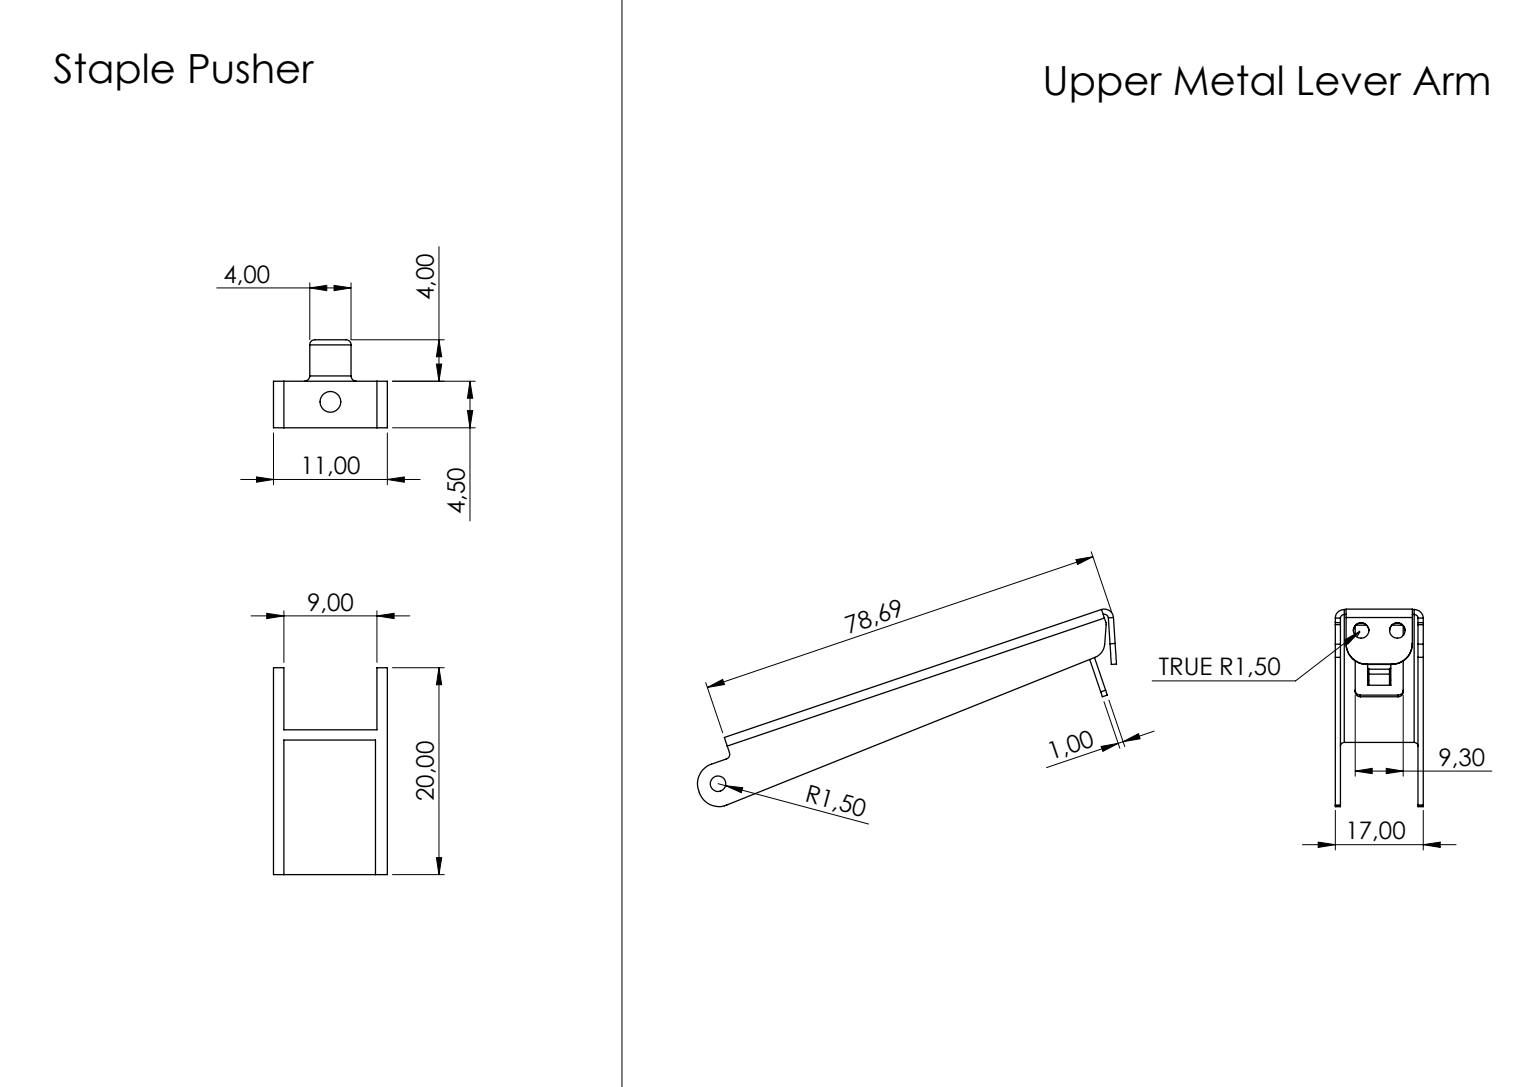
ISO-10303-21;
HEADER;
FILE_DESCRIPTION (('STEP AP214'),
    '1' );
FILE_NAME ('Staple Pusher.step',
    '2026-10-06T10:23:46',
    ( '' ),
    ( '' ),
    'SwSTEP 2.0',
    'SolidWorks 2020',
    '' );
FILE_SCHEMA (( 'AUTOMOTIVE_DESIGN' ));
ENDSEC;

DATA;
#63=ORIENTED_EDGE ( 'NONE', *, *, #7607, .F. ) ;
#105=( NAMED_UNIT ( * ) PLANE_ANGLE_UNIT ( ) SI_UNIT ( $, .RADIAN. ) );
#123=ADVANCED_FACE ( 'NONE', ( #785 ), #7110, .F. ) ;
#143=VECTOR ( 'NONE', #19074, 1000.000000000000000 ) ;
#190=ORIENTED_EDGE ( 'NONE', *, *, #18404, .F. ) ;
#193=DIRECTION ( 'NONE',  ( -1.927470528863119788E-16, -1.000000000000000000, 2.999999999999999839E-15 ) ) ;
#203=VERTEX_POINT ( 'NONE', #23192 ) ;
#209=LINE ( 'NONE', #23668, #17662 ) ;
#231=EDGE_CURVE ( 'NONE', #16465, #14577, #22942, .T. ) ;
#236=CARTESIAN_POINT ( 'NONE',  ( 40.81606138205700063, 9.191238522346999673, 69.30501292736997243 ) ) ;
#250=EDGE_CURVE ( 'NONE', #6034, #3058, #21270, .T. ) ;
#262=CARTESIAN_POINT ( 'NONE',  ( 32.81606138205700773, 2.191238522347013440, 73.80501292737000085 ) ) ;
#307=ORIENTED_EDGE ( 'NONE', *, *, #22779, .T. ) ;
#351=FACE_OUTER_BOUND ( 'NONE', #1891, .T. ) ;
#379=DIRECTION ( 'NONE',  ( 1.000000000000000000, 0.000000000000000000, 0.000000000000000000 ) ) ;
#383=AXIS2_PLACEMENT_3D ( 'NONE', #20572, #5122, #2903 ) ;
#385=CARTESIAN_POINT ( 'NONE',  ( 36.81606138205700063, 8.691238522346987239, 65.30501292736998664 ) ) ;
#404=EDGE_LOOP ( 'NONE', ( #18442, #12105, #307, #7710 ) ) ;
#415=ORIENTED_EDGE ( 'NONE', *, *, #6576, .T. ) ;
#419=CYLINDRICAL_SURFACE ( 'NONE', #8765, 0.5000000000000004441 ) ;
#442=ORIENTED_EDGE ( 'NONE', *, *, #7387, .T. ) ;
#462=DIRECTION ( 'NONE',  ( 1.000000000000000000, 3.614007241618344826E-17, -1.084202172485503317E-31 ) ) ;
#467=VERTEX_POINT ( 'NONE', #6689 ) ;
#486=PLANE ( 'NONE',  #5925 ) ;
#553=DIRECTION ( 'NONE',  ( 0.000000000000000000, 2.999999999999999839E-15, 1.000000000000000000 ) ) ;
#562=VERTEX_POINT ( 'NONE', #2686 ) ;
#577=ADVANCED_FACE ( 'NONE', ( #16345 ), #8767, .F. ) ;
#593=EDGE_CURVE ( 'NONE', #5442, #4334, #1137, .T. ) ;
#621=ORIENTED_EDGE ( 'NONE', *, *, #6367, .T. ) ;
#629=EDGE_LOOP ( 'NONE', ( #17511, #10756, #22625, #6939, #1629, #11779, #9994, #21905 ) ) ;
#650=EDGE_CURVE ( 'NONE', #5870, #848, #10535, .T. ) ;
#674=VECTOR ( 'NONE', #14592, 1000.000000000000000 ) ;
#690=CARTESIAN_POINT ( 'NONE',  ( 32.81606138205700773, 2.191238522347000117, 69.30501292737000085 ) ) ;
#728=DIRECTION ( 'NONE',  ( 0.000000000000000000, -1.000000000000000000, 2.999999999999999839E-15 ) ) ;
#732=( BOUNDED_CURVE ( )  B_SPLINE_CURVE ( 3, ( #2177, #11606, #21769, #236 ),
 .UNSPECIFIED., .F., .T. ) 
 B_SPLINE_CURVE_WITH_KNOTS ( ( 4, 4 ),
 ( 0.000000000000000000, 1.570796326794895004 ),
 .UNSPECIFIED. ) 
 CURVE ( )  GEOMETRIC_REPRESENTATION_ITEM ( )  RATIONAL_B_SPLINE_CURVE ( ( 1.000000000000000000, 0.8047378541243649375, 0.8047378541243649375, 1.000000000000000000 ) ) 
 REPRESENTATION_ITEM ( '' )  );
#761=CARTESIAN_POINT ( 'NONE',  ( 33.81606138205700063, 22.19123852234703520, 80.30501292736994401 ) ) ;
#785=FACE_OUTER_BOUND ( 'NONE', #18859, .T. ) ;
#797=VECTOR ( 'NONE', #6910, 1000.000000000000000 ) ;
#823=CARTESIAN_POINT ( 'NONE',  ( 36.31606138205700063, 8.691238522346989015, 65.80501292736998664 ) ) ;
#843=CARTESIAN_POINT ( 'NONE',  ( 40.31606138205700063, 8.691238522346987239, 65.30501292736998664 ) ) ;
#848=VERTEX_POINT ( 'NONE', #18891 ) ;
#858=DIRECTION ( 'NONE',  ( 0.000000000000000000, 2.999999999999999839E-15, 1.000000000000000000 ) ) ;
#900=EDGE_CURVE ( 'NONE', #13184, #17478, #14637, .T. ) ;
#904=VECTOR ( 'NONE', #2124, 1000.000000000000000 ) ;
#912=ADVANCED_FACE ( 'NONE', ( #16562 ), #11803, .T. ) ;
#927=LINE ( 'NONE', #12805, #16343 ) ;
#964=AXIS2_PLACEMENT_3D ( 'NONE', #21763, #4252, #7865 ) ;
#974=ORIENTED_EDGE ( 'NONE', *, *, #19644, .F. ) ;
#1000=VECTOR ( 'NONE', #20638, 1000.000000000000000 ) ;
#1001=CARTESIAN_POINT ( 'NONE',  ( 35.81606138205700063, 9.191238522346999673, 69.30501292736997243 ) ) ;
#1007=ORIENTED_EDGE ( 'NONE', *, *, #15153, .F. ) ;
#1092=EDGE_CURVE ( 'NONE', #467, #5442, #24144, .T. ) ;
#1096=DIRECTION ( 'NONE',  ( 0.000000000000000000, 1.000000000000000000, -2.999999999999999839E-15 ) ) ;
#1134=CARTESIAN_POINT ( 'NONE',  ( 33.81606138205700063, 15.19123852234700323, 70.30501292736995822 ) ) ;
#1137=LINE ( 'NONE', #2653, #13495 ) ;
#1179=DIRECTION ( 'NONE',  ( 0.000000000000000000, 1.000000000000000000, -2.999999999999999839E-15 ) ) ;
#1184=ADVANCED_FACE ( 'NONE', ( #6400 ), #19925, .T. ) ;
#1216=EDGE_LOOP ( 'NONE', ( #10411, #24861, #10562, #15495, #17319, #20995, #18206, #9644 ) ) ;
#1217=VECTOR ( 'NONE', #3864, 1000.000000000000000 ) ;
#1267=ORIENTED_EDGE ( 'NONE', *, *, #5167, .T. ) ;
#1275=ADVANCED_FACE ( 'NONE', ( #8845 ), #16686, .F. ) ;
#1303=ORIENTED_EDGE ( 'NONE', *, *, #4139, .F. ) ;
#1313=ORIENTED_EDGE ( 'NONE', *, *, #19104, .T. ) ;
#1337=CARTESIAN_POINT ( 'NONE',  ( 32.81606138205700773, 2.191238522347013440, 73.80501292737000085 ) ) ;
#1365=CARTESIAN_POINT ( 'NONE',  ( 32.81606138205700773, 2.191238522347013440, 73.80501292737000085 ) ) ;
#1435=LINE ( 'NONE', #16906, #1000 ) ;
#1489=EDGE_LOOP ( 'NONE', ( #16805, #24401, #621, #24675, #16930 ) ) ;
#1492=CARTESIAN_POINT ( 'NONE',  ( 42.81606138205700063, 16.19123852234703520, 80.30501292736995822 ) ) ;
#1496=PLANE ( 'NONE',  #16992 ) ;
#1569=ORIENTED_EDGE ( 'NONE', *, *, #14152, .T. ) ;
#1629=ORIENTED_EDGE ( 'NONE', *, *, #3717, .T. ) ;
#1678=SURFACE_STYLE_FILL_AREA ( #9947 ) ;
#1738=DIRECTION ( 'NONE',  ( 0.000000000000000000, -2.999999999999999839E-15, -1.000000000000000000 ) ) ;
#1805=ADVANCED_FACE ( 'NONE', ( #22575 ), #20906, .F. ) ;
#1829=ORIENTED_EDGE ( 'NONE', *, *, #2608, .T. ) ;
#1839=ORIENTED_EDGE ( 'NONE', *, *, #24052, .F. ) ;
#1853=ORIENTED_EDGE ( 'NONE', *, *, #1903, .F. ) ;
#1891=EDGE_LOOP ( 'NONE', ( #16584, #9694, #23122, #20814 ) ) ;
#1903=EDGE_CURVE ( 'NONE', #12694, #9681, #8685, .T. ) ;
#1906=EDGE_CURVE ( 'NONE', #10160, #8707, #24745, .T. ) ;
#1911=CARTESIAN_POINT ( 'NONE',  ( 36.31606138205700063, 5.691238522346989903, 65.80501292736998664 ) ) ;
#1930=CARTESIAN_POINT ( 'NONE',  ( 32.81606138205700773, 2.191238522347013440, 73.80501292737000085 ) ) ;
#1936=PRESENTATION_STYLE_ASSIGNMENT (( #13426 ) ) ;
#1981=DIRECTION ( 'NONE',  ( 1.000000000000000000, 0.000000000000000000, -0.000000000000000000 ) ) ;
#1983=EDGE_LOOP ( 'NONE', ( #14043, #19238, #19687, #25097 ) ) ;
#1986=VERTEX_POINT ( 'NONE', #25119 ) ;
#1996=CARTESIAN_POINT ( 'NONE',  ( 38.31606138205700063, 15.19123852234700323, 70.30501292736995822 ) ) ;
#1998=DIRECTION ( 'NONE',  ( 0.000000000000000000, -2.999999999999999839E-15, -1.000000000000000000 ) ) ;
#2000=AXIS2_PLACEMENT_3D ( 'NONE', #9286, #12766, #22537 ) ;
#2012=CARTESIAN_POINT ( 'NONE',  ( 32.81606138205700773, 22.19123852234701388, 73.80501292736992980 ) ) ;
#2015=DIRECTION ( 'NONE',  ( -1.000000000000000000, 0.000000000000000000, 0.000000000000000000 ) ) ;
#2044=PLANE ( 'NONE',  #16388 ) ;
#2052=ORIENTED_EDGE ( 'NONE', *, *, #22004, .F. ) ;
#2059=EDGE_LOOP ( 'NONE', ( #10504, #1303, #7748, #10759, #1267 ) ) ;
#2102=CARTESIAN_POINT ( 'NONE',  ( 36.10895460087045450, 5.484131741160450879, 69.30501292736998664 ) ) ;
#2109=MECHANICAL_DESIGN_GEOMETRIC_PRESENTATION_REPRESENTATION('',(#21879),#6646);
#2124=DIRECTION ( 'NONE',  ( 1.000000000000000000, 0.000000000000000000, -0.000000000000000000 ) ) ;
#2141=FACE_OUTER_BOUND ( 'NONE', #11810, .T. ) ;
#2173=CARTESIAN_POINT ( 'NONE',  ( 43.81606138205700063, 8.191238522346990791, 65.80501292736998664 ) ) ;
#2177=CARTESIAN_POINT ( 'NONE',  ( 40.31606138205700063, 8.691238522346997897, 68.80501292736998664 ) ) ;
#2184=EDGE_CURVE ( 'NONE', #4421, #25070, #3535, .T. ) ;
#2217=CARTESIAN_POINT ( 'NONE',  ( 40.52316816324353965, 5.484131741160450879, 69.30501292736998664 ) ) ;
#2224=LINE ( 'NONE', #4423, #8434 ) ;
#2261=DIRECTION ( 'NONE',  ( 1.000000000000000000, 0.000000000000000000, 0.000000000000000000 ) ) ;
#2293=SURFACE_STYLE_FILL_AREA ( #20953 ) ;
#2315=DIRECTION ( 'NONE',  ( 0.000000000000000000, 1.000000000000000000, -2.999999999999999839E-15 ) ) ;
#2317=CARTESIAN_POINT ( 'NONE',  ( 36.31606138205699352, 8.691238522346996120, 69.09790614618343341 ) ) ;
#2323=CARTESIAN_POINT ( 'NONE',  ( 36.81606138205700063, 6.191238522346988127, 65.30501292736998664 ) ) ;
#2333=DIRECTION ( 'NONE',  ( 0.000000000000000000, 1.000000000000000000, -2.999999999999999839E-15 ) ) ;
#2397=PLANE ( 'NONE',  #13514 ) ;
#2404=EDGE_CURVE ( 'NONE', #6235, #17478, #14094, .T. ) ;
#2443=AXIS2_PLACEMENT_3D ( 'NONE', #4060, #8182, #10241 ) ;
#2510=DIRECTION ( 'NONE',  ( 0.000000000000000000, -2.999999999999999839E-15, -1.000000000000000000 ) ) ;
#2577=DIRECTION ( 'NONE',  ( 1.000000000000000000, 0.000000000000000000, -0.000000000000000000 ) ) ;
#2608=EDGE_CURVE ( 'NONE', #9423, #562, #927, .T. ) ;
#2622=VECTOR ( 'NONE', #19427, 1000.000000000000000 ) ;
#2627=CARTESIAN_POINT ( 'NONE',  ( 36.31606138205699352, 8.691238522346985462, 65.51211970855652567 ) ) ;
#2652=CARTESIAN_POINT ( 'NONE',  ( 36.31606138205700063, 9.191238522346999673, 69.30501292736997243 ) ) ;
#2653=CARTESIAN_POINT ( 'NONE',  ( 32.81606138205700773, 22.19123852234699967, 69.30501292736994401 ) ) ;
#2686=CARTESIAN_POINT ( 'NONE',  ( 40.31606138205700063, 8.691238522346989015, 65.80501292736998664 ) ) ;
#2694=CARTESIAN_POINT ( 'NONE',  ( 42.68042513965293949, 15.19123852234701388, 73.80501292736995822 ) ) ;
#2711=ORIENTED_EDGE ( 'NONE', *, *, #14927, .F. ) ;
#2724=VERTEX_POINT ( 'NONE', #15354 ) ;
#2742=CARTESIAN_POINT ( 'NONE',  ( 36.31606138205700063, 8.691238522346989015, 65.80501292736998664 ) ) ;
#2771=VECTOR ( 'NONE', #18659, 1000.000000000000000 ) ;
#2782=CARTESIAN_POINT ( 'NONE',  ( 36.31606138205700063, 5.691238522346988127, 65.30501292736998664 ) ) ;
#2812=CARTESIAN_POINT ( 'NONE',  ( 32.81606138205700773, 22.19123852234699967, 69.30501292736994401 ) ) ;
#2866=CIRCLE ( 'NONE', #6186, 1.000000000000000888 ) ;
#2900=ORIENTED_EDGE ( 'NONE', *, *, #21220, .T. ) ;
#2903=DIRECTION ( 'NONE',  ( 1.000000000000000000, 0.000000000000000000, 0.000000000000000000 ) ) ;
#2928=VERTEX_POINT ( 'NONE', #2323 ) ;
#2967=ORIENTED_EDGE ( 'NONE', *, *, #1092, .T. ) ;
#3033=CARTESIAN_POINT ( 'NONE',  ( 33.81606138205700063, 22.19123852234699967, 69.30501292736994401 ) ) ;
#3035=FACE_OUTER_BOUND ( 'NONE', #20986, .T. ) ;
#3058=VERTEX_POINT ( 'NONE', #8642 ) ;
#3146=CARTESIAN_POINT ( 'NONE',  ( 40.31606138205700773, 8.691238522346985462, 65.51211970855652567 ) ) ;
#3205=EDGE_CURVE ( 'NONE', #848, #2928, #20946, .T. ) ;
#3237=VECTOR ( 'NONE', #3931, 1000.000000000000000 ) ;
#3248=DIRECTION ( 'NONE',  ( 0.000000000000000000, 1.000000000000000000, -2.999999999999999839E-15 ) ) ;
#3279=DIRECTION ( 'NONE',  ( -1.956963323498894821E-16, 1.000000000000000000, -2.999999999999999839E-15 ) ) ;
#3295=( NAMED_UNIT ( * ) PLANE_ANGLE_UNIT ( ) SI_UNIT ( $, .RADIAN. ) );
#3314=VERTEX_POINT ( 'NONE', #19072 ) ;
#3331=LINE ( 'NONE', #5532, #19828 ) ;
#3347=AXIS2_PLACEMENT_3D ( 'NONE', #20363, #2315, #379 ) ;
#3356=EDGE_LOOP ( 'NONE', ( #23510, #24602, #16175, #23690 ) ) ;
#3385=CARTESIAN_POINT ( 'NONE',  ( 33.81606138205700063, 2.191238522347003226, 70.30501292737000085 ) ) ;
#3409=ADVANCED_FACE ( 'NONE', ( #12370 ), #2044, .F. ) ;
#3425=DIRECTION ( 'NONE',  ( 0.000000000000000000, 2.999999999999999839E-15, 1.000000000000000000 ) ) ;
#3438=PLANE ( 'NONE',  #4644 ) ;
#3449=LINE ( 'NONE', #13494, #11858 ) ;
#3509=CARTESIAN_POINT ( 'NONE',  ( 42.81606138205700063, 22.19123852234699967, 69.30501292736994401 ) ) ;
#3535=LINE ( 'NONE', #5478, #22502 ) ;
#3540=CARTESIAN_POINT ( 'NONE',  ( 42.81606138205700063, 2.191238522347013884, 73.80501292737000085 ) ) ;
#3568=VECTOR ( 'NONE', #24239, 1000.000000000000000 ) ;
#3583=CARTESIAN_POINT ( 'NONE',  ( 43.81606138205700063, 2.191238522347000117, 69.30501292737000085 ) ) ;
#3680=ORIENTED_EDGE ( 'NONE', *, *, #9929, .F. ) ;
#3703=ORIENTED_EDGE ( 'NONE', *, *, #9232, .T. ) ;
#3717=EDGE_CURVE ( 'NONE', #5857, #7071, #209, .T. ) ;
#3739=CARTESIAN_POINT ( 'NONE',  ( 43.81606138205700063, 2.191238522346988127, 65.30501292737000085 ) ) ;
#3748=FILL_AREA_STYLE_COLOUR ( '', #14877 ) ;
#3829=DIRECTION ( 'NONE',  ( 0.000000000000000000, 2.999999999999999839E-15, 1.000000000000000000 ) ) ;
#3864=DIRECTION ( 'NONE',  ( 1.927470528863119788E-16, 1.000000000000000000, -2.999999999999999839E-15 ) ) ;
#3876=APPLICATION_CONTEXT ( 'automotive_design' ) ;
#3931=DIRECTION ( 'NONE',  ( 1.000000000000000000, 0.000000000000000000, -0.000000000000000000 ) ) ;
#3986=DIRECTION ( 'NONE',  ( 0.000000000000000000, 1.000000000000000000, -2.999999999999999839E-15 ) ) ;
#4021=VECTOR ( 'NONE', #6407, 1000.000000000000000 ) ;
#4039=VECTOR ( 'NONE', #8852, 1000.000000000000000 ) ;
#4060=CARTESIAN_POINT ( 'NONE',  ( 40.31606138205700063, 9.191238522346997897, 68.80501292736998664 ) ) ;
#4121=( NAMED_UNIT ( * ) SI_UNIT ( $, .STERADIAN. ) SOLID_ANGLE_UNIT ( ) );
#4131=ORIENTED_EDGE ( 'NONE', *, *, #2404, .F. ) ;
#4139=EDGE_CURVE ( 'NONE', #15007, #21826, #25055, .T. ) ;
#4153=EDGE_CURVE ( 'NONE', #8707, #4754, #8867, .T. ) ;
#4155=PLANE ( 'NONE',  #12494 ) ;
#4173=CARTESIAN_POINT ( 'NONE',  ( 42.68042513965293949, 2.191238522347003226, 70.30501292737000085 ) ) ;
#4180=CARTESIAN_POINT ( 'NONE',  ( 36.31606138205700063, 5.691238522346998785, 68.80501292736998664 ) ) ;
#4252=DIRECTION ( 'NONE',  ( 0.000000000000000000, 2.999999999999999839E-15, 1.000000000000000000 ) ) ;
#4282=EDGE_CURVE ( 'NONE', #19015, #5870, #21143, .T. ) ;
#4334=VERTEX_POINT ( 'NONE', #14111 ) ;
#4356=ORIENTED_EDGE ( 'NONE', *, *, #22779, .F. ) ;
#4373=CARTESIAN_POINT ( 'NONE',  ( 33.81606138205700063, 2.191238522347003226, 70.30501292737000085 ) ) ;
#4377=CARTESIAN_POINT ( 'NONE',  ( 42.68042513965293949, 2.191238522347003226, 70.30501292737000085 ) ) ;
#4411=DIRECTION ( 'NONE',  ( 1.000000000000000000, 0.000000000000000000, 0.000000000000000000 ) ) ;
#4421=VERTEX_POINT ( 'NONE', #18601 ) ;
#4423=CARTESIAN_POINT ( 'NONE',  ( 33.81606138205700063, 15.19123852234701388, 73.80501292736995822 ) ) ;
#4473=CARTESIAN_POINT ( 'NONE',  ( 40.31606138205700063, 8.691238522346987239, 65.30501292736998664 ) ) ;
#4478=CARTESIAN_POINT ( 'NONE',  ( 42.81606138205700063, 22.19123852234703520, 80.30501292736994401 ) ) ;
#4484=ORIENTED_EDGE ( 'NONE', *, *, #14301, .F. ) ;
#4491=VECTOR ( 'NONE', #11130, 1000.000000000000000 ) ;
#4500=LINE ( 'NONE', #4377, #9031 ) ;
#4524=VECTOR ( 'NONE', #9145, 1000.000000000000000 ) ;
#4553=DIRECTION ( 'NONE',  ( 1.000000000000000000, 0.000000000000000000, -0.000000000000000000 ) ) ;
#4556=AXIS2_PLACEMENT_3D ( 'NONE', #21742, #12479, #6415 ) ;
#4644=AXIS2_PLACEMENT_3D ( 'NONE', #1492, #193, #1738 ) ;
#4683=ORIENTED_EDGE ( 'NONE', *, *, #18404, .T. ) ;
#4733=ORIENTED_EDGE ( 'NONE', *, *, #2184, .F. ) ;
#4754=VERTEX_POINT ( 'NONE', #12164 ) ;
#4768=EDGE_CURVE ( 'NONE', #13664, #17658, #23623, .T. ) ;
#4773=LINE ( 'NONE', #10717, #17444 ) ;
#4798=DIRECTION ( 'NONE',  ( 0.000000000000000000, -2.999999999999999839E-15, -1.000000000000000000 ) ) ;
#4867=CARTESIAN_POINT ( 'NONE',  ( 32.81606138205700773, 22.19123852234699967, 69.30501292736994401 ) ) ;
#4892=VERTEX_POINT ( 'NONE', #22564 ) ;
#4902=DIRECTION ( 'NONE',  ( 0.000000000000000000, -2.999999999999999839E-15, -1.000000000000000000 ) ) ;
#4963=CARTESIAN_POINT ( 'NONE',  ( 40.31606138205700063, 8.691238522346989015, 65.80501292736998664 ) ) ;
#5122=DIRECTION ( 'NONE',  ( 0.000000000000000000, 1.000000000000000000, -2.999999999999999839E-15 ) ) ;
#5130=AXIS2_PLACEMENT_3D ( 'NONE', #11785, #4553, #8421 ) ;
#5139=LINE ( 'NONE', #12749, #22298 ) ;
#5144=CARTESIAN_POINT ( 'NONE',  ( 32.81606138205700773, 22.19123852234701388, 73.80501292736992980 ) ) ;
#5166=ADVANCED_FACE ( 'NONE', ( #25104 ), #13541, .T. ) ;
#5167=EDGE_CURVE ( 'NONE', #22981, #13614, #2866, .T. ) ;
#5180=ORIENTED_EDGE ( 'NONE', *, *, #250, .T. ) ;
#5193=FACE_OUTER_BOUND ( 'NONE', #629, .T. ) ;
#5270=CARTESIAN_POINT ( 'NONE',  ( 40.31606138205700063, 5.191238522346999673, 69.30501292736998664 ) ) ;
#5397=UNCERTAINTY_MEASURE_WITH_UNIT (LENGTH_MEASURE( 1.000000000000000082E-05 ), #23294, 'distance_accuracy_value', 'NONE');
#5398=VECTOR ( 'NONE', #19032, 1000.000000000000000 ) ;
#5442=VERTEX_POINT ( 'NONE', #20474 ) ;
#5478=CARTESIAN_POINT ( 'NONE',  ( 32.81606138205700773, 16.19123852234701388, 73.80501292736995822 ) ) ;
#5485=EDGE_CURVE ( 'NONE', #6235, #15007, #12886, .T. ) ;
#5532=CARTESIAN_POINT ( 'NONE',  ( 33.81606138205700063, 2.191238522347013440, 73.80501292737000085 ) ) ;
#5623=EDGE_LOOP ( 'NONE', ( #15814, #4131, #21557, #25354 ) ) ;
#5631=FACE_OUTER_BOUND ( 'NONE', #13241, .T. ) ;
#5660=SURFACE_STYLE_USAGE ( .BOTH. , #25348 ) ;
#5661=CARTESIAN_POINT ( 'NONE',  ( 36.81606138205700063, 6.191238522346988127, 65.30501292736998664 ) ) ;
#5687=( NAMED_UNIT ( * ) PLANE_ANGLE_UNIT ( ) SI_UNIT ( $, .RADIAN. ) );
#5797=CARTESIAN_POINT ( 'NONE',  ( 42.68042513965293949, 2.191238522347013440, 73.80501292737000085 ) ) ;
#5844=PLANE ( 'NONE',  #5130 ) ;
#5857=VERTEX_POINT ( 'NONE', #690 ) ;
#5870=VERTEX_POINT ( 'NONE', #823 ) ;
#5886=LINE ( 'NONE', #7693, #23529 ) ;
#5925=AXIS2_PLACEMENT_3D ( 'NONE', #7171, #13095, #20823 ) ;
#5970=ORIENTED_EDGE ( 'NONE', *, *, #6000, .T. ) ;
#6000=EDGE_CURVE ( 'NONE', #10377, #3314, #16803, .T. ) ;
#6029=APPLICATION_CONTEXT ( 'automotive_design' ) ;
#6034=VERTEX_POINT ( 'NONE', #1337 ) ;
#6115=EDGE_LOOP ( 'NONE', ( #3703, #4356, #24721, #1853 ) ) ;
#6118=CARTESIAN_POINT ( 'NONE',  ( 42.81606138205700063, 16.19123852234703520, 80.30501292736995822 ) ) ;
#6137=LINE ( 'NONE', #24019, #24716 ) ;
#6141=CARTESIAN_POINT ( 'NONE',  ( 33.81606138205700063, 15.19123852234700323, 70.30501292736995822 ) ) ;
#6142=DIRECTION ( 'NONE',  ( 0.000000000000000000, -1.000000000000000000, 0.000000000000000000 ) ) ;
#6150=LINE ( 'NONE', #4473, #4021 ) ;
#6186=AXIS2_PLACEMENT_3D ( 'NONE', #23576, #21649, #11878 ) ;
#6188=ADVANCED_FACE ( 'NONE', ( #23480 ), #5844, .F. ) ;
#6202=DIRECTION ( 'NONE',  ( 0.000000000000000000, -1.000000000000000000, 2.999999999999999839E-15 ) ) ;
#6235=VERTEX_POINT ( 'NONE', #20134 ) ;
#6319=EDGE_CURVE ( 'NONE', #17478, #203, #2224, .T. ) ;
#6331=DIRECTION ( 'NONE',  ( 0.000000000000000000, -1.000000000000000000, 2.999999999999999839E-15 ) ) ;
#6367=EDGE_CURVE ( 'NONE', #13507, #6369, #1435, .T. ) ;
#6369=VERTEX_POINT ( 'NONE', #22568 ) ;
#6389=ORIENTED_EDGE ( 'NONE', *, *, #3205, .T. ) ;
#6400=FACE_OUTER_BOUND ( 'NONE', #10407, .T. ) ;
#6407=DIRECTION ( 'NONE',  ( 0.000000000000000000, 2.999999999999999839E-15, 1.000000000000000000 ) ) ;
#6415=DIRECTION ( 'NONE',  ( -1.445602896647339903E-16, 1.000000000000000000, -2.999999999999999839E-15 ) ) ;
#6416=EDGE_LOOP ( 'NONE', ( #15821, #22360, #20683, #13474 ) ) ;
#6455=CARTESIAN_POINT ( 'NONE',  ( 35.81606138205700063, 9.191238522346999673, 69.30501292736997243 ) ) ;
#6465=VECTOR ( 'NONE', #2510, 1000.000000000000000 ) ;
#6493=FACE_OUTER_BOUND ( 'NONE', #11204, .T. ) ;
#6518=ORIENTED_EDGE ( 'NONE', *, *, #16824, .F. ) ;
#6576=EDGE_CURVE ( 'NONE', #6034, #10160, #13422, .T. ) ;
#6646=( GEOMETRIC_REPRESENTATION_CONTEXT ( 3 ) GLOBAL_UNCERTAINTY_ASSIGNED_CONTEXT ( ( #16158 ) ) GLOBAL_UNIT_ASSIGNED_CONTEXT ( ( #25249, #5687, #23585 ) ) REPRESENTATION_CONTEXT ( 'NONE', 'WORKASPACE' ) );
#6647=LINE ( 'NONE', #14382, #6913 ) ;
#6655=VECTOR ( 'NONE', #13137, 1000.000000000000000 ) ;
#6689=CARTESIAN_POINT ( 'NONE',  ( 42.81606138205700063, 22.19123852234701388, 73.80501292736992980 ) ) ;
#6697=CARTESIAN_POINT ( 'NONE',  ( 36.81606138205700063, 2.191238522346989903, 65.80501292737000085 ) ) ;
#6771=ADVANCED_BREP_SHAPE_REPRESENTATION ( '', ( #17330, #2000 ), #23998 ) ;
#6894=DIRECTION ( 'NONE',  ( -1.000000000000000000, -1.956963323498894821E-16, 5.870889970496684443E-31 ) ) ;
#6910=DIRECTION ( 'NONE',  ( 0.000000000000000000, 1.000000000000000000, -2.999999999999999839E-15 ) ) ;
#6913=VECTOR ( 'NONE', #14508, 1000.000000000000000 ) ;
#6917=ORIENTED_EDGE ( 'NONE', *, *, #7387, .F. ) ;
#6924=EDGE_LOOP ( 'NONE', ( #11359, #2052 ) ) ;
#6928=EDGE_CURVE ( 'NONE', #13507, #203, #13012, .T. ) ;
#6939=ORIENTED_EDGE ( 'NONE', *, *, #18851, .F. ) ;
#6941=CARTESIAN_POINT ( 'NONE',  ( 40.31606138205700773, 5.691238522346986350, 65.51211970855653988 ) ) ;
#7016=DIRECTION ( 'NONE',  ( 0.000000000000000000, 1.000000000000000000, -2.999999999999999839E-15 ) ) ;
#7071=VERTEX_POINT ( 'NONE', #15696 ) ;
#7110=CYLINDRICAL_SURFACE ( 'NONE', #16342, 0.4999999999999995559 ) ;
#7171=CARTESIAN_POINT ( 'NONE',  ( 32.81606138205700773, 22.19123852234699967, 69.30501292736994401 ) ) ;
#7233=DIRECTION ( 'NONE',  ( 0.000000000000000000, 1.000000000000000000, -2.999999999999999839E-15 ) ) ;
#7244=CARTESIAN_POINT ( 'NONE',  ( 40.81606138205700063, 8.691238522346999673, 69.30501292736998664 ) ) ;
#7252=VECTOR ( 'NONE', #24084, 1000.000000000000000 ) ;
#7264=ORIENTED_EDGE ( 'NONE', *, *, #4282, .T. ) ;
#7300=DIRECTION ( 'NONE',  ( 1.000000000000000000, 0.000000000000000000, -0.000000000000000000 ) ) ;
#7316=CLOSED_SHELL ( 'NONE', ( #21757, #912, #6188, #1275, #3409, #12132, #123, #21257, #11449, #9745, #1184, #13040, #8158, #5166, #24270, #17690, #19312, #24499, #19394, #14924, #1805, #12499, #9959, #577, #12730, #8926, #13194, #13060, #17434 ) ) ;
#7387=EDGE_CURVE ( 'NONE', #203, #3058, #16579, .T. ) ;
#7391=LINE ( 'NONE', #3385, #4491 ) ;
#7607=EDGE_CURVE ( 'NONE', #4892, #2928, #5886, .T. ) ;
#7693=CARTESIAN_POINT ( 'NONE',  ( 36.31606138205700063, 6.191238522346988127, 65.30501292736998664 ) ) ;
#7710=ORIENTED_EDGE ( 'NONE', *, *, #17518, .T. ) ;
#7748=ORIENTED_EDGE ( 'NONE', *, *, #7774, .F. ) ;
#7764=PRODUCT_CONTEXT ( 'NONE', #3876, 'mechanical' ) ;
#7774=EDGE_CURVE ( 'NONE', #17636, #15007, #10383, .T. ) ;
#7820=CARTESIAN_POINT ( 'NONE',  ( 37.31606138205700063, 12.69123852234700678, 71.30501292736997243 ) ) ;
#7864=CARTESIAN_POINT ( 'NONE',  ( 36.31606138205699352, 5.691238522346986350, 65.51211970855653988 ) ) ;
#7865=DIRECTION ( 'NONE',  ( 1.000000000000000000, 0.000000000000000000, -0.000000000000000000 ) ) ;
#8058=EDGE_LOOP ( 'NONE', ( #22523, #13290, #11880, #4484 ) ) ;
#8110=AXIS2_PLACEMENT_3D ( 'NONE', #19995, #2333, #4411 ) ;
#8158=ADVANCED_FACE ( 'NONE', ( #12524 ), #23829, .T. ) ;
#8182=DIRECTION ( 'NONE',  ( -1.000000000000000000, 0.000000000000000000, 0.000000000000000000 ) ) ;
#8202=DIRECTION ( 'NONE',  ( 1.000000000000000000, 0.000000000000000000, -0.000000000000000000 ) ) ;
#8305=DIRECTION ( 'NONE',  ( 1.000000000000000000, 0.000000000000000000, 0.000000000000000000 ) ) ;
#8336=ORIENTED_EDGE ( 'NONE', *, *, #6319, .F. ) ;
#8353=PLANE ( 'NONE',  #18198 ) ;
#8397=LINE ( 'NONE', #16239, #7252 ) ;
#8414=ORIENTED_EDGE ( 'NONE', *, *, #17520, .T. ) ;
#8421=DIRECTION ( 'NONE',  ( 0.000000000000000000, 2.999999999999999839E-15, 1.000000000000000000 ) ) ;
#8434=VECTOR ( 'NONE', #10102, 1000.000000000000000 ) ;
#8435=CARTESIAN_POINT ( 'NONE',  ( 40.81606138205700063, 5.691238522346998785, 68.80501292736998664 ) ) ;
#8533=CARTESIAN_POINT ( 'NONE',  ( 37.31606138205700063, 15.19123852234700500, 71.30501292736995822 ) ) ;
#8541=DIRECTION ( 'NONE',  ( 0.000000000000000000, 1.000000000000000000, -2.999999999999999839E-15 ) ) ;
#8642=CARTESIAN_POINT ( 'NONE',  ( 33.81606138205700063, 2.191238522347013440, 73.80501292737000085 ) ) ;
#8660=VECTOR ( 'NONE', #25232, 1000.000000000000000 ) ;
#8685=LINE ( 'NONE', #16915, #674 ) ;
#8707=VERTEX_POINT ( 'NONE', #4867 ) ;
#8750=CARTESIAN_POINT ( 'NONE',  ( 40.31606138205700063, 5.691238522346988127, 65.30501292736998664 ) ) ;
#8765=AXIS2_PLACEMENT_3D ( 'NONE', #8435, #20021, #8305 ) ;
#8767=PLANE ( 'NONE',  #11032 ) ;
#8808=AXIS2_PLACEMENT_3D ( 'NONE', #2173, #11739, #23809 ) ;
#8845=FACE_OUTER_BOUND ( 'NONE', #10900, .T. ) ;
#8852=DIRECTION ( 'NONE',  ( 0.000000000000000000, -2.999999999999999839E-15, -1.000000000000000000 ) ) ;
#8857=LINE ( 'NONE', #3033, #797 ) ;
#8867=LINE ( 'NONE', #20831, #17679 ) ;
#8913=ORIENTED_EDGE ( 'NONE', *, *, #1092, .F. ) ;
#8926=ADVANCED_FACE ( 'NONE', ( #5193 ), #13051, .F. ) ;
#8943=LINE ( 'NONE', #14353, #25032 ) ;
#8981=DIRECTION ( 'NONE',  ( -1.000000000000000000, 0.000000000000000000, 0.000000000000000000 ) ) ;
#8985=DIRECTION ( 'NONE',  ( 0.000000000000000000, -2.999999999999999839E-15, -1.000000000000000000 ) ) ;
#9031=VECTOR ( 'NONE', #20083, 1000.000000000000000 ) ;
#9099=CARTESIAN_POINT ( 'NONE',  ( 40.10895460087045450, 8.484131741160446438, 65.30501292736998664 ) ) ;
#9141=CARTESIAN_POINT ( 'NONE',  ( 36.81606138205700063, 8.191238522346989015, 65.30501292736998664 ) ) ;
#9145=DIRECTION ( 'NONE',  ( 1.000000000000000000, 0.000000000000000000, -0.000000000000000000 ) ) ;
#9232=EDGE_CURVE ( 'NONE', #12694, #22231, #24566, .T. ) ;
#9264=EDGE_CURVE ( 'NONE', #562, #5870, #8397, .T. ) ;
#9286=CARTESIAN_POINT ( 'NONE',  ( 0.000000000000000000, 0.000000000000000000, 0.000000000000000000 ) ) ;
#9423=VERTEX_POINT ( 'NONE', #16615 ) ;
#9567=VECTOR ( 'NONE', #23708, 1000.000000000000000 ) ;
#9636=CARTESIAN_POINT ( 'NONE',  ( 32.81606138205700773, 22.19123852234701388, 73.80501292736992980 ) ) ;
#9640=MECHANICAL_DESIGN_GEOMETRIC_PRESENTATION_REPRESENTATION('',(#17438),#12526);
#9644=ORIENTED_EDGE ( 'NONE', *, *, #15572, .F. ) ;
#9652=PLANE ( 'NONE',  #10635 ) ;
#9653=PRODUCT_DEFINITION ( 'UNKNOWN', '', #23210, #16222 ) ;
#9681=VERTEX_POINT ( 'NONE', #20078 ) ;
#9694=ORIENTED_EDGE ( 'NONE', *, *, #2608, .F. ) ;
#9705=PLANE ( 'NONE',  #18258 ) ;
#9745=ADVANCED_FACE ( 'NONE', ( #351 ), #10164, .T. ) ;
#9814=DIRECTION ( 'NONE',  ( 1.000000000000000000, 0.000000000000000000, -0.000000000000000000 ) ) ;
#9897=CYLINDRICAL_SURFACE ( 'NONE', #14910, 0.5000000000000004441 ) ;
#9929=EDGE_CURVE ( 'NONE', #848, #9423, #23141, .T. ) ;
#9947=FILL_AREA_STYLE ('',( #3748 ) ) ;
#9959=ADVANCED_FACE ( 'NONE', ( #5631 ), #1496, .T. ) ;
#9963=VECTOR ( 'NONE', #6331, 1000.000000000000000 ) ;
#9994=ORIENTED_EDGE ( 'NONE', *, *, #17987, .F. ) ;
#10024=DIRECTION ( 'NONE',  ( 0.000000000000000000, 2.999999999999999839E-15, 1.000000000000000000 ) ) ;
#10097=CARTESIAN_POINT ( 'NONE',  ( 40.31606138205700063, 5.691238522346998785, 68.80501292736998664 ) ) ;
#10102=DIRECTION ( 'NONE',  ( -1.000000000000000000, -1.956963323498894821E-16, 5.870889970496684443E-31 ) ) ;
#10131=DIRECTION ( 'NONE',  ( 0.000000000000000000, 1.000000000000000000, -2.999999999999999839E-15 ) ) ;
#10160=VERTEX_POINT ( 'NONE', #2012 ) ;
#10164=CYLINDRICAL_SURFACE ( 'NONE', #20689, 0.5000000000000004441 ) ;
#10208=VECTOR ( 'NONE', #11060, 1000.000000000000000 ) ;
#10239=LINE ( 'NONE', #6118, #16453 ) ;
#10241=DIRECTION ( 'NONE',  ( 0.000000000000000000, 1.000000000000000000, 0.000000000000000000 ) ) ;
#10368=ORIENTED_EDGE ( 'NONE', *, *, #9264, .T. ) ;
#10377=VERTEX_POINT ( 'NONE', #14875 ) ;
#10383=CIRCLE ( 'NONE', #19021, 1.000000000000000888 ) ;
#10391=ORIENTED_EDGE ( 'NONE', *, *, #1906, .T. ) ;
#10407=EDGE_LOOP ( 'NONE', ( #6389, #63, #1839, #3680 ) ) ;
#10411=ORIENTED_EDGE ( 'NONE', *, *, #4153, .T. ) ;
#10414=LINE ( 'NONE', #2782, #18194 ) ;
#10433=COLOUR_RGB ( '', 0.66274510, 0.83137255, 0.94901961) ;
#10489=ORIENTED_EDGE ( 'NONE', *, *, #18787, .F. ) ;
#10504=ORIENTED_EDGE ( 'NONE', *, *, #24901, .F. ) ;
#10519=CARTESIAN_POINT ( 'NONE',  ( 42.81606138205700063, 22.19123852234703520, 80.30501292736994401 ) ) ;
#10535=LINE ( 'NONE', #18012, #14714 ) ;
#10536=FACE_OUTER_BOUND ( 'NONE', #20667, .T. ) ;
#10562=ORIENTED_EDGE ( 'NONE', *, *, #231, .F. ) ;
#10573=AXIS2_PLACEMENT_3D ( 'NONE', #23899, #8202, #6142 ) ;
#10594=VECTOR ( 'NONE', #7300, 1000.000000000000000 ) ;
#10635=AXIS2_PLACEMENT_3D ( 'NONE', #25326, #21481, #3829 ) ;
#10716=EDGE_CURVE ( 'NONE', #20891, #19678, #13098, .T. ) ;
#10717=CARTESIAN_POINT ( 'NONE',  ( 33.81606138205700063, 2.191238522347003226, 70.30501292737000085 ) ) ;
#10730=DIRECTION ( 'NONE',  ( 1.000000000000000000, 0.000000000000000000, -0.000000000000000000 ) ) ;
#10756=ORIENTED_EDGE ( 'NONE', *, *, #20283, .T. ) ;
#10759=ORIENTED_EDGE ( 'NONE', *, *, #20936, .T. ) ;
#10804=LINE ( 'NONE', #8750, #2771 ) ;
#10824=VECTOR ( 'NONE', #12040, 1000.000000000000000 ) ;
#10900=EDGE_LOOP ( 'NONE', ( #21455, #23238, #1569, #20821, #12695, #19741, #21236, #24698 ) ) ;
#10912=PLANE ( 'NONE',  #11573 ) ;
#10951=ORIENTED_EDGE ( 'NONE', *, *, #25045, .T. ) ;
#10965=ORIENTED_EDGE ( 'NONE', *, *, #15849, .F. ) ;
#11032=AXIS2_PLACEMENT_3D ( 'NONE', #2812, #18673, #16604 ) ;
#11034=DIRECTION ( 'NONE',  ( 0.000000000000000000, 1.000000000000000000, -2.999999999999999839E-15 ) ) ;
#11060=DIRECTION ( 'NONE',  ( 0.000000000000000000, 1.000000000000000000, -2.999999999999999839E-15 ) ) ;
#11130=DIRECTION ( 'NONE',  ( 0.000000000000000000, 2.999999999999999839E-15, 1.000000000000000000 ) ) ;
#11204=EDGE_LOOP ( 'NONE', ( #19772, #10965, #13766, #190 ) ) ;
#11224=LINE ( 'NONE', #22806, #143 ) ;
#11310=EDGE_CURVE ( 'NONE', #5870, #12694, #5139, .T. ) ;
#11323=DIRECTION ( 'NONE',  ( 0.000000000000000000, 1.000000000000000000, -2.999999999999999839E-15 ) ) ;
#11351=FACE_OUTER_BOUND ( 'NONE', #11483, .T. ) ;
#11359=ORIENTED_EDGE ( 'NONE', *, *, #5167, .F. ) ;
#11382=DIRECTION ( 'NONE',  ( 3.614007241618344826E-17, -1.000000000000000000, 2.999999999999999839E-15 ) ) ;
#11449=ADVANCED_FACE ( 'NONE', ( #11708 ), #9897, .F. ) ;
#11483=EDGE_LOOP ( 'NONE', ( #7264, #24776, #6518, #11621 ) ) ;
#11485=LINE ( 'NONE', #13409, #23037 ) ;
#11573=AXIS2_PLACEMENT_3D ( 'NONE', #18764, #1096, #8985 ) ;
#11606=CARTESIAN_POINT ( 'NONE',  ( 40.31606138205700773, 8.691238522346996120, 69.09790614618343341 ) ) ;
#11619=DIRECTION ( 'NONE',  ( -1.000000000000000000, 1.927470528863119788E-16, -5.782411586589358909E-31 ) ) ;
#11621=ORIENTED_EDGE ( 'NONE', *, *, #19958, .F. ) ;
#11679=CARTESIAN_POINT ( 'NONE',  ( 39.31606138205700063, 16.19123852234700678, 71.30501292736995822 ) ) ;
#11705=DIRECTION ( 'NONE',  ( -1.000000000000000000, 0.000000000000000000, 0.000000000000000000 ) ) ;
#11708=FACE_OUTER_BOUND ( 'NONE', #22440, .T. ) ;
#11717=ORIENTED_EDGE ( 'NONE', *, *, #7607, .T. ) ;
#11739=DIRECTION ( 'NONE',  ( -1.000000000000000000, 0.000000000000000000, 0.000000000000000000 ) ) ;
#11755=ORIENTED_EDGE ( 'NONE', *, *, #14287, .F. ) ;
#11779=ORIENTED_EDGE ( 'NONE', *, *, #20081, .T. ) ;
#11785=CARTESIAN_POINT ( 'NONE',  ( 42.68042513965293949, 2.191238522347003226, 70.30501292737000085 ) ) ;
#11803=PLANE ( 'NONE',  #20865 ) ;
#11810=EDGE_LOOP ( 'NONE', ( #2967, #20673, #13703, #974 ) ) ;
#11836=VECTOR ( 'NONE', #11034, 1000.000000000000000 ) ;
#11840=EDGE_LOOP ( 'NONE', ( #16477, #24634, #10489, #4733 ) ) ;
#11858=VECTOR ( 'NONE', #16983, 1000.000000000000000 ) ;
#11878=DIRECTION ( 'NONE',  ( 1.000000000000000000, 0.000000000000000000, 0.000000000000000000 ) ) ;
#11880=ORIENTED_EDGE ( 'NONE', *, *, #17520, .F. ) ;
#11998=LINE ( 'NONE', #13661, #1217 ) ;
#12032=ORIENTED_EDGE ( 'NONE', *, *, #18714, .T. ) ;
#12040=DIRECTION ( 'NONE',  ( 0.000000000000000000, 2.999999999999999839E-15, 1.000000000000000000 ) ) ;
#12047=EDGE_LOOP ( 'NONE', ( #21140, #8913, #14740, #10951 ) ) ;
#12105=ORIENTED_EDGE ( 'NONE', *, *, #15849, .T. ) ;
#12120=VECTOR ( 'NONE', #7016, 1000.000000000000000 ) ;
#12132=ADVANCED_FACE ( 'NONE', ( #6493 ), #419, .F. ) ;
#12159=CYLINDRICAL_SURFACE ( 'NONE', #8110, 1.000000000000000888 ) ;
#12164=CARTESIAN_POINT ( 'NONE',  ( 33.81606138205700063, 22.19123852234699967, 69.30501292736994401 ) ) ;
#12218=PLANE ( 'NONE',  #4556 ) ;
#12219=ORIENTED_EDGE ( 'NONE', *, *, #18983, .T. ) ;
#12224=DIRECTION ( 'NONE',  ( 0.000000000000000000, 2.999999999999999839E-15, 1.000000000000000000 ) ) ;
#12308=DIRECTION ( 'NONE',  ( 0.000000000000000000, -2.999999999999999839E-15, -1.000000000000000000 ) ) ;
#12329=CARTESIAN_POINT ( 'NONE',  ( 33.81606138205700063, 16.19123852234701388, 73.80501292736995822 ) ) ;
#12370=FACE_OUTER_BOUND ( 'NONE', #15620, .T. ) ;
#12409=ORIENTED_EDGE ( 'NONE', *, *, #19958, .T. ) ;
#12439=EDGE_CURVE ( 'NONE', #5442, #16465, #17556, .T. ) ;
#12479=DIRECTION ( 'NONE',  ( -1.000000000000000000, -1.445602896647339903E-16, 4.336808689942019400E-31 ) ) ;
#12494=AXIS2_PLACEMENT_3D ( 'NONE', #262, #4902, #16360 ) ;
#12499=ADVANCED_FACE ( 'NONE', ( #21168 ), #9705, .F. ) ;
#12524=FACE_OUTER_BOUND ( 'NONE', #3356, .T. ) ;
#12526=( GEOMETRIC_REPRESENTATION_CONTEXT ( 3 ) GLOBAL_UNCERTAINTY_ASSIGNED_CONTEXT ( ( #5397 ) ) GLOBAL_UNIT_ASSIGNED_CONTEXT ( ( #23294, #105, #4121 ) ) REPRESENTATION_CONTEXT ( 'NONE', 'WORKASPACE' ) );
#12579=CARTESIAN_POINT ( 'NONE',  ( 37.31606138205700063, 16.19123852234700678, 71.30501292736995822 ) ) ;
#12673=CARTESIAN_POINT ( 'NONE',  ( 38.31606138205700063, 15.19123852234700500, 71.30501292736995822 ) ) ;
#12694=VERTEX_POINT ( 'NONE', #23966 ) ;
#12695=ORIENTED_EDGE ( 'NONE', *, *, #5485, .F. ) ;
#12730=ADVANCED_FACE ( 'NONE', ( #13940 ), #4155, .F. ) ;
#12749=CARTESIAN_POINT ( 'NONE',  ( 36.31606138205700063, 8.691238522346987239, 65.30501292736998664 ) ) ;
#12757=CARTESIAN_POINT ( 'NONE',  ( 40.31606138205700063, 5.691238522346989903, 65.80501292736998664 ) ) ;
#12766=DIRECTION ( 'NONE',  ( 0.000000000000000000, 0.000000000000000000, 1.000000000000000000 ) ) ;
#12805=CARTESIAN_POINT ( 'NONE',  ( 40.31606138205700063, 8.691238522346989015, 65.80501292736998664 ) ) ;
#12866=EDGE_CURVE ( 'NONE', #6369, #16802, #4773, .T. ) ;
#12886=LINE ( 'NONE', #1134, #24293 ) ;
#12977=CARTESIAN_POINT ( 'NONE',  ( 42.68042513965293949, 2.191238522347013440, 73.80501292737000085 ) ) ;
#13012=LINE ( 'NONE', #14553, #21207 ) ;
#13023=EDGE_CURVE ( 'NONE', #15007, #13507, #11224, .T. ) ;
#13040=ADVANCED_FACE ( 'NONE', ( #11351 ), #15954, .T. ) ;
#13051=PLANE ( 'NONE',  #18405 ) ;
#13060=ADVANCED_FACE ( 'NONE', ( #15575, #21892 ), #15833, .F. ) ;
#13095=DIRECTION ( 'NONE',  ( 0.000000000000000000, -1.000000000000000000, 2.999999999999999839E-15 ) ) ;
#13098=( BOUNDED_CURVE ( )  B_SPLINE_CURVE ( 3, ( #19761, #2102, #17844, #4180 ),
 .UNSPECIFIED., .F., .T. ) 
 B_SPLINE_CURVE_WITH_KNOTS ( ( 4, 4 ),
 ( 1.570796326794895004, 3.141592653589795336 ),
 .UNSPECIFIED. ) 
 CURVE ( )  GEOMETRIC_REPRESENTATION_ITEM ( )  RATIONAL_B_SPLINE_CURVE ( ( 1.000000000000000000, 0.8047378541243649375, 0.8047378541243649375, 1.000000000000000000 ) ) 
 REPRESENTATION_ITEM ( '' )  );
#13137=DIRECTION ( 'NONE',  ( 1.000000000000000000, 0.000000000000000000, -0.000000000000000000 ) ) ;
#13184=VERTEX_POINT ( 'NONE', #5797 ) ;
#13186=DIRECTION ( 'NONE',  ( -1.445602896647339903E-16, 1.000000000000000000, -2.999999999999999839E-15 ) ) ;
#13194=ADVANCED_FACE ( 'NONE', ( #17527 ), #486, .F. ) ;
#13206=ORIENTED_EDGE ( 'NONE', *, *, #23492, .T. ) ;
#13232=( LENGTH_UNIT ( ) NAMED_UNIT ( * ) SI_UNIT ( .MILLI., .METRE. ) );
#13241=EDGE_LOOP ( 'NONE', ( #25082, #415, #10391, #23792 ) ) ;
#13242=FACE_OUTER_BOUND ( 'NONE', #11840, .T. ) ;
#13278=VECTOR ( 'NONE', #10131, 1000.000000000000000 ) ;
#13290=ORIENTED_EDGE ( 'NONE', *, *, #22858, .T. ) ;
#13390=ORIENTED_EDGE ( 'NONE', *, *, #11310, .T. ) ;
#13409=CARTESIAN_POINT ( 'NONE',  ( 39.81606138205699352, 5.691238522346988127, 65.30501292736998664 ) ) ;
#13422=LINE ( 'NONE', #17671, #20772 ) ;
#13426=SURFACE_STYLE_USAGE ( .BOTH. , #15600 ) ;
#13444=ORIENTED_EDGE ( 'NONE', *, *, #6367, .F. ) ;
#13468=LINE ( 'NONE', #3540, #19686 ) ;
#13474=ORIENTED_EDGE ( 'NONE', *, *, #6000, .F. ) ;
#13494=CARTESIAN_POINT ( 'NONE',  ( 40.31606138205700063, 5.691238522346998785, 68.80501292736998664 ) ) ;
#13495=VECTOR ( 'NONE', #20189, 1000.000000000000000 ) ;
#13496=CARTESIAN_POINT ( 'NONE',  ( 35.81606138205700063, 5.691238522346998785, 68.80501292736998664 ) ) ;
#13507=VERTEX_POINT ( 'NONE', #6141 ) ;
#13514=AXIS2_PLACEMENT_3D ( 'NONE', #4478, #462, #10024 ) ;
#13541=PLANE ( 'NONE',  #14007 ) ;
#13562=VECTOR ( 'NONE', #8981, 1000.000000000000000 ) ;
#13614=VERTEX_POINT ( 'NONE', #12579 ) ;
#13624=DIRECTION ( 'NONE',  ( 1.000000000000000000, 0.000000000000000000, -0.000000000000000000 ) ) ;
#13661=CARTESIAN_POINT ( 'NONE',  ( 39.31606138205700063, 12.69123852234700678, 71.30501292736997243 ) ) ;
#13664=VERTEX_POINT ( 'NONE', #20294 ) ;
#13703=ORIENTED_EDGE ( 'NONE', *, *, #23212, .F. ) ;
#13766=ORIENTED_EDGE ( 'NONE', *, *, #4768, .T. ) ;
#13940=FACE_OUTER_BOUND ( 'NONE', #19367, .T. ) ;
#14007=AXIS2_PLACEMENT_3D ( 'NONE', #3739, #15724, #15211 ) ;
#14034=PRESENTATION_STYLE_ASSIGNMENT (( #5660 ) ) ;
#14043=ORIENTED_EDGE ( 'NONE', *, *, #14152, .F. ) ;
#14094=LINE ( 'NONE', #18219, #3568 ) ;
#14111=CARTESIAN_POINT ( 'NONE',  ( 43.81606138205700063, 22.19123852234699967, 69.30501292736994401 ) ) ;
#14152=EDGE_CURVE ( 'NONE', #21826, #17636, #17834, .T. ) ;
#14221=DIRECTION ( 'NONE',  ( 0.000000000000000000, -1.000000000000000000, 2.999999999999999839E-15 ) ) ;
#14287=EDGE_CURVE ( 'NONE', #20891, #13664, #19299, .T. ) ;
#14291=ORIENTED_EDGE ( 'NONE', *, *, #14301, .T. ) ;
#14301=EDGE_CURVE ( 'NONE', #25070, #2724, #3331, .T. ) ;
#14330=CARTESIAN_POINT ( 'NONE',  ( 40.31606138205700773, 5.691238522346996120, 69.09790614618344762 ) ) ;
#14353=CARTESIAN_POINT ( 'NONE',  ( 43.81606138205700063, 2.191238522347000117, 69.30501292737000085 ) ) ;
#14382=CARTESIAN_POINT ( 'NONE',  ( 32.81606138205700773, 2.191238522347000117, 69.30501292737000085 ) ) ;
#14460=ORIENTED_EDGE ( 'NONE', *, *, #14600, .T. ) ;
#14491=ORIENTED_EDGE ( 'NONE', *, *, #9232, .F. ) ;
#14508=DIRECTION ( 'NONE',  ( 0.000000000000000000, 2.999999999999999839E-15, 1.000000000000000000 ) ) ;
#14553=CARTESIAN_POINT ( 'NONE',  ( 33.81606138205700063, 15.19123852234700323, 70.30501292736995822 ) ) ;
#14577=VERTEX_POINT ( 'NONE', #20331 ) ;
#14592=DIRECTION ( 'NONE',  ( 1.000000000000000000, 0.000000000000000000, -0.000000000000000000 ) ) ;
#14600=EDGE_CURVE ( 'NONE', #848, #19678, #10414, .T. ) ;
#14620=ORIENTED_EDGE ( 'NONE', *, *, #11310, .F. ) ;
#14637=LINE ( 'NONE', #12977, #11836 ) ;
#14670=DIRECTION ( 'NONE',  ( 0.000000000000000000, 2.999999999999999839E-15, 1.000000000000000000 ) ) ;
#14714=VECTOR ( 'NONE', #22114, 1000.000000000000000 ) ;
#14740=ORIENTED_EDGE ( 'NONE', *, *, #14927, .T. ) ;
#14772=DIRECTION ( 'NONE',  ( 1.000000000000000000, 0.000000000000000000, -0.000000000000000000 ) ) ;
#14874=ORIENTED_EDGE ( 'NONE', *, *, #10716, .T. ) ;
#14875=CARTESIAN_POINT ( 'NONE',  ( 43.81606138205700063, 2.191238522347013440, 73.80501292737000085 ) ) ;
#14877=COLOUR_RGB ( '', 0.66274510, 0.83137255, 0.94901961) ;
#14910=AXIS2_PLACEMENT_3D ( 'NONE', #13496, #21228, #2015 ) ;
#14924=ADVANCED_FACE ( 'NONE', ( #21093, #13242 ), #3438, .F. ) ;
#14927=EDGE_CURVE ( 'NONE', #467, #3314, #23512, .T. ) ;
#14958=CARTESIAN_POINT ( 'NONE',  ( 38.31606138205700063, 16.19123852234700678, 71.30501292736995822 ) ) ;
#15007=VERTEX_POINT ( 'NONE', #1996 ) ;
#15139=ORIENTED_EDGE ( 'NONE', *, *, #18714, .F. ) ;
#15153=EDGE_CURVE ( 'NONE', #19678, #12694, #20038, .T. ) ;
#15174=CARTESIAN_POINT ( 'NONE',  ( 39.81606138205699352, 6.191238522346988127, 65.30501292736998664 ) ) ;
#15211=DIRECTION ( 'NONE',  ( 0.000000000000000000, 1.000000000000000000, -2.999999999999999839E-15 ) ) ;
#15228=AXIS2_PLACEMENT_3D ( 'NONE', #6697, #6202, #18430 ) ;
#15230=SHAPE_DEFINITION_REPRESENTATION ( #17966, #15514 ) ;
#15331=LINE ( 'NONE', #23567, #8660 ) ;
#15354=CARTESIAN_POINT ( 'NONE',  ( 33.81606138205700063, 22.19123852234701388, 73.80501292736992980 ) ) ;
#15417=DIRECTION ( 'NONE',  ( -1.000000000000000000, -1.956963323498894821E-16, 5.870889970496684443E-31 ) ) ;
#15495=ORIENTED_EDGE ( 'NONE', *, *, #12439, .F. ) ;
#15514=SHAPE_REPRESENTATION ( 'Staple Pusher', ( #2000 ), #23998 ) ;
#15523=ORIENTED_EDGE ( 'NONE', *, *, #4153, .F. ) ;
#15539=DIRECTION ( 'NONE',  ( -1.000000000000000000, 0.000000000000000000, 0.000000000000000000 ) ) ;
#15572=EDGE_CURVE ( 'NONE', #8707, #5857, #20260, .T. ) ;
#15575=FACE_BOUND ( 'NONE', #404, .T. ) ;
#15583=ORIENTED_EDGE ( 'NONE', *, *, #17987, .T. ) ;
#15600=SURFACE_SIDE_STYLE ('',( #1678 ) ) ;
#15620=EDGE_LOOP ( 'NONE', ( #442, #18018, #13444, #19517 ) ) ;
#15631=EDGE_CURVE ( 'NONE', #16802, #13184, #16261, .T. ) ;
#15694=FILL_AREA_STYLE_COLOUR ( '', #10433 ) ;
#15696=CARTESIAN_POINT ( 'NONE',  ( 43.81606138205700063, 2.191238522347000117, 69.30501292737000085 ) ) ;
#15724=DIRECTION ( 'NONE',  ( 0.000000000000000000, -2.999999999999999839E-15, -1.000000000000000000 ) ) ;
#15814=ORIENTED_EDGE ( 'NONE', *, *, #900, .T. ) ;
#15821=ORIENTED_EDGE ( 'NONE', *, *, #20081, .F. ) ;
#15833=PLANE ( 'NONE',  #964 ) ;
#15849=EDGE_CURVE ( 'NONE', #13664, #22879, #22694, .T. ) ;
#15954=CYLINDRICAL_SURFACE ( 'NONE', #8808, 0.5000000000000004441 ) ;
#16080=DIRECTION ( 'NONE',  ( -1.445602896647339903E-16, 1.000000000000000000, -2.999999999999999839E-15 ) ) ;
#16107=CARTESIAN_POINT ( 'NONE',  ( 36.31606138205700063, 8.691238522346997897, 68.80501292736998664 ) ) ;
#16127=DIRECTION ( 'NONE',  ( 1.000000000000000000, 0.000000000000000000, 0.000000000000000000 ) ) ;
#16158=UNCERTAINTY_MEASURE_WITH_UNIT (LENGTH_MEASURE( 1.000000000000000082E-05 ), #25249, 'distance_accuracy_value', 'NONE');
#16175=ORIENTED_EDGE ( 'NONE', *, *, #4282, .F. ) ;
#16222=PRODUCT_DEFINITION_CONTEXT ( 'detailed design', #6029, 'design' ) ;
#16239=CARTESIAN_POINT ( 'NONE',  ( 36.31606138205700063, 8.691238522346989015, 65.80501292736998664 ) ) ;
#16261=LINE ( 'NONE', #4173, #10824 ) ;
#16342=AXIS2_PLACEMENT_3D ( 'NONE', #20896, #10730, #20385 ) ;
#16343=VECTOR ( 'NONE', #13186, 1000.000000000000000 ) ;
#16345=FACE_OUTER_BOUND ( 'NONE', #12047, .T. ) ;
#16360=DIRECTION ( 'NONE',  ( 0.000000000000000000, 1.000000000000000000, -2.999999999999999839E-15 ) ) ;
#16388=AXIS2_PLACEMENT_3D ( 'NONE', #4373, #23933, #3986 ) ;
#16416=CARTESIAN_POINT ( 'NONE',  ( 36.31606138205700063, 8.691238522346997897, 68.80501292736998664 ) ) ;
#16434=CARTESIAN_POINT ( 'NONE',  ( 40.81606138205700063, 9.191238522346999673, 69.30501292736997243 ) ) ;
#16453=VECTOR ( 'NONE', #12308, 1000.000000000000000 ) ;
#16465=VERTEX_POINT ( 'NONE', #17643 ) ;
#16477=ORIENTED_EDGE ( 'NONE', *, *, #23212, .T. ) ;
#16489=( BOUNDED_CURVE ( )  B_SPLINE_CURVE ( 3, ( #12757, #6941, #19052, #15174 ),
 .UNSPECIFIED., .F., .T. ) 
 B_SPLINE_CURVE_WITH_KNOTS ( ( 4, 4 ),
 ( 0.000000000000000000, 1.570796326794895004 ),
 .UNSPECIFIED. ) 
 CURVE ( )  GEOMETRIC_REPRESENTATION_ITEM ( )  RATIONAL_B_SPLINE_CURVE ( ( 1.000000000000000000, 0.8047378541243649375, 0.8047378541243649375, 1.000000000000000000 ) ) 
 REPRESENTATION_ITEM ( '' )  );
#16508=EDGE_CURVE ( 'NONE', #4334, #7071, #23162, .T. ) ;
#16549=CARTESIAN_POINT ( 'NONE',  ( 33.81606138205700063, 15.19123852234700323, 70.30501292736995822 ) ) ;
#16562=FACE_OUTER_BOUND ( 'NONE', #1489, .T. ) ;
#16579=LINE ( 'NONE', #20454, #17810 ) ;
#16584=ORIENTED_EDGE ( 'NONE', *, *, #16824, .T. ) ;
#16604=DIRECTION ( 'NONE',  ( -1.000000000000000000, 0.000000000000000000, 0.000000000000000000 ) ) ;
#16615=CARTESIAN_POINT ( 'NONE',  ( 40.31606138205700063, 5.691238522346989903, 65.80501292736998664 ) ) ;
#16686=PLANE ( 'NONE',  #22098 ) ;
#16769=DIRECTION ( 'NONE',  ( -1.445602896647339903E-16, 1.000000000000000000, -2.999999999999999839E-15 ) ) ;
#16802=VERTEX_POINT ( 'NONE', #16809 ) ;
#16803=LINE ( 'NONE', #24636, #12120 ) ;
#16805=ORIENTED_EDGE ( 'NONE', *, *, #5485, .T. ) ;
#16809=CARTESIAN_POINT ( 'NONE',  ( 42.68042513965293949, 2.191238522347003226, 70.30501292737000085 ) ) ;
#16815=ORIENTED_EDGE ( 'NONE', *, *, #1903, .T. ) ;
#16824=EDGE_CURVE ( 'NONE', #1986, #562, #17334, .T. ) ;
#16906=CARTESIAN_POINT ( 'NONE',  ( 33.81606138205700063, 2.191238522347003226, 70.30501292737000085 ) ) ;
#16915=CARTESIAN_POINT ( 'NONE',  ( 40.31606138205700063, 8.691238522346997897, 68.80501292736998664 ) ) ;
#16930=ORIENTED_EDGE ( 'NONE', *, *, #22175, .T. ) ;
#16983=DIRECTION ( 'NONE',  ( 1.445602896647339903E-16, -1.000000000000000000, 2.999999999999999839E-15 ) ) ;
#16992=AXIS2_PLACEMENT_3D ( 'NONE', #21224, #11705, #11323 ) ;
#17005=VECTOR ( 'NONE', #14221, 1000.000000000000000 ) ;
#17009=CARTESIAN_POINT ( 'NONE',  ( 39.31606138205700063, 15.19123852234700500, 71.30501292736995822 ) ) ;
#17128=DIRECTION ( 'NONE',  ( 0.000000000000000000, 1.000000000000000000, -2.999999999999999839E-15 ) ) ;
#17210=DIRECTION ( 'NONE',  ( 3.614007241618344826E-17, -1.000000000000000000, 2.999999999999999839E-15 ) ) ;
#17319=ORIENTED_EDGE ( 'NONE', *, *, #593, .T. ) ;
#17330=MANIFOLD_SOLID_BREP ( 'NONE', #7316 ) ;
#17334=( BOUNDED_CURVE ( )  B_SPLINE_CURVE ( 3, ( #24518, #9099, #3146, #4963 ),
 .UNSPECIFIED., .F., .T. ) 
 B_SPLINE_CURVE_WITH_KNOTS ( ( 4, 4 ),
 ( 1.570796326794895004, 3.141592653589795336 ),
 .UNSPECIFIED. ) 
 CURVE ( )  GEOMETRIC_REPRESENTATION_ITEM ( )  RATIONAL_B_SPLINE_CURVE ( ( 1.000000000000000000, 0.8047378541243649375, 0.8047378541243649375, 1.000000000000000000 ) ) 
 REPRESENTATION_ITEM ( '' )  );
#17434=ADVANCED_FACE ( 'NONE', ( #24082 ), #23831, .F. ) ;
#17438=STYLED_ITEM ( 'NONE', ( #14034 ), #6771 ) ;
#17444=VECTOR ( 'NONE', #2577, 1000.000000000000000 ) ;
#17478=VERTEX_POINT ( 'NONE', #2694 ) ;
#17502=FACE_OUTER_BOUND ( 'NONE', #23990, .T. ) ;
#17511=ORIENTED_EDGE ( 'NONE', *, *, #12866, .F. ) ;
#17518=EDGE_CURVE ( 'NONE', #22231, #20891, #18431, .T. ) ;
#17520=EDGE_CURVE ( 'NONE', #2724, #4754, #18313, .T. ) ;
#17527=FACE_OUTER_BOUND ( 'NONE', #19189, .T. ) ;
#17556=LINE ( 'NONE', #3509, #24386 ) ;
#17624=AXIS2_PLACEMENT_3D ( 'NONE', #24364, #24484, #1179 ) ;
#17636=VERTEX_POINT ( 'NONE', #17009 ) ;
#17643=CARTESIAN_POINT ( 'NONE',  ( 42.81606138205700063, 16.19123852234699967, 69.30501292736995822 ) ) ;
#17658=VERTEX_POINT ( 'NONE', #22417 ) ;
#17662=VECTOR ( 'NONE', #23910, 1000.000000000000000 ) ;
#17671=CARTESIAN_POINT ( 'NONE',  ( 32.81606138205700773, 2.191238522347013440, 73.80501292737000085 ) ) ;
#17677=DIRECTION ( 'NONE',  ( 0.000000000000000000, -2.999999999999999839E-15, -1.000000000000000000 ) ) ;
#17679=VECTOR ( 'NONE', #14772, 1000.000000000000000 ) ;
#17688=FACE_OUTER_BOUND ( 'NONE', #2059, .T. ) ;
#17690=ADVANCED_FACE ( 'NONE', ( #22002 ), #8353, .F. ) ;
#17713=ORIENTED_EDGE ( 'NONE', *, *, #10716, .F. ) ;
#17715=DIRECTION ( 'NONE',  ( -1.000000000000000000, 1.927470528863119788E-16, -5.782411586589358909E-31 ) ) ;
#17810=VECTOR ( 'NONE', #728, 1000.000000000000000 ) ;
#17834=CIRCLE ( 'NONE', #21117, 1.000000000000000888 ) ;
#17844=CARTESIAN_POINT ( 'NONE',  ( 36.31606138205699352, 5.691238522346996120, 69.09790614618344762 ) ) ;
#17851=CARTESIAN_POINT ( 'NONE',  ( 40.31606138205700063, 8.191238522346989015, 65.30501292736998664 ) ) ;
#17966=PRODUCT_DEFINITION_SHAPE ( 'NONE', 'NONE',  #9653 ) ;
#17987=EDGE_CURVE ( 'NONE', #13184, #10377, #19026, .T. ) ;
#18010=VECTOR ( 'NONE', #11619, 1000.000000000000000 ) ;
#18012=CARTESIAN_POINT ( 'NONE',  ( 36.31606138205700063, 5.691238522346989903, 65.80501292736998664 ) ) ;
#18018=ORIENTED_EDGE ( 'NONE', *, *, #20283, .F. ) ;
#18032=CARTESIAN_POINT ( 'NONE',  ( 39.81606138205699352, 2.191238522346989015, 65.80501292737000085 ) ) ;
#18109=CYLINDRICAL_SURFACE ( 'NONE', #2443, 0.5000000000000004441 ) ;
#18194=VECTOR ( 'NONE', #12224, 1000.000000000000000 ) ;
#18198=AXIS2_PLACEMENT_3D ( 'NONE', #843, #20443, #24419 ) ;
#18204=CARTESIAN_POINT ( 'NONE',  ( 38.31606138205700063, 15.19123852234700500, 71.30501292736995822 ) ) ;
#18206=ORIENTED_EDGE ( 'NONE', *, *, #3717, .F. ) ;
#18219=CARTESIAN_POINT ( 'NONE',  ( 42.68042513965293949, 15.19123852234700323, 70.30501292736995822 ) ) ;
#18257=CARTESIAN_POINT ( 'NONE',  ( 33.81606138205700063, 16.19123852234703520, 80.30501292736995822 ) ) ;
#18258=AXIS2_PLACEMENT_3D ( 'NONE', #22964, #24877, #3248 ) ;
#18313=LINE ( 'NONE', #761, #9567 ) ;
#18376=LINE ( 'NONE', #18257, #4039 ) ;
#18404=EDGE_CURVE ( 'NONE', #9681, #17658, #3449, .T. ) ;
#18405=AXIS2_PLACEMENT_3D ( 'NONE', #20904, #21660, #17677 ) ;
#18430=DIRECTION ( 'NONE',  ( -1.000000000000000000, 0.000000000000000000, 0.000000000000000000 ) ) ;
#18431=LINE ( 'NONE', #20108, #9963 ) ;
#18442=ORIENTED_EDGE ( 'NONE', *, *, #14287, .T. ) ;
#18531=LINE ( 'NONE', #385, #10208 ) ;
#18601=CARTESIAN_POINT ( 'NONE',  ( 42.81606138205700063, 16.19123852234701388, 73.80501292736995822 ) ) ;
#18643=ORIENTED_EDGE ( 'NONE', *, *, #9929, .T. ) ;
#18659=DIRECTION ( 'NONE',  ( 0.000000000000000000, 2.999999999999999839E-15, 1.000000000000000000 ) ) ;
#18673=DIRECTION ( 'NONE',  ( 0.000000000000000000, -1.000000000000000000, 2.999999999999999839E-15 ) ) ;
#18714=EDGE_CURVE ( 'NONE', #562, #9681, #6150, .T. ) ;
#18764=CARTESIAN_POINT ( 'NONE',  ( 40.31606138205700063, 5.691238522346988127, 65.30501292736998664 ) ) ;
#18787=EDGE_CURVE ( 'NONE', #25070, #14577, #18376, .T. ) ;
#18851=EDGE_CURVE ( 'NONE', #5857, #6034, #6647, .T. ) ;
#18859=EDGE_LOOP ( 'NONE', ( #14874, #22019, #19012, #11755 ) ) ;
#18891=CARTESIAN_POINT ( 'NONE',  ( 36.31606138205700063, 5.691238522346989903, 65.80501292736998664 ) ) ;
#18983=EDGE_CURVE ( 'NONE', #2928, #19015, #18531, .T. ) ;
#19012=ORIENTED_EDGE ( 'NONE', *, *, #4768, .F. ) ;
#19015=VERTEX_POINT ( 'NONE', #9141 ) ;
#19021=AXIS2_PLACEMENT_3D ( 'NONE', #12673, #23775, #2261 ) ;
#19026=LINE ( 'NONE', #1365, #10594 ) ;
#19032=DIRECTION ( 'NONE',  ( 1.927470528863119788E-16, 1.000000000000000000, -2.999999999999999839E-15 ) ) ;
#19052=CARTESIAN_POINT ( 'NONE',  ( 40.10895460087045450, 5.898345303533535144, 65.30501292737000085 ) ) ;
#19055=UNCERTAINTY_MEASURE_WITH_UNIT (LENGTH_MEASURE( 1.000000000000000082E-05 ), #13232, 'distance_accuracy_value', 'NONE');
#19072=CARTESIAN_POINT ( 'NONE',  ( 43.81606138205700063, 22.19123852234701388, 73.80501292736992980 ) ) ;
#19074=DIRECTION ( 'NONE',  ( -1.000000000000000000, -1.956963323498894821E-16, 5.870889970496684443E-31 ) ) ;
#19085=DIRECTION ( 'NONE',  ( 1.000000000000000000, 0.000000000000000000, 0.000000000000000000 ) ) ;
#19104=EDGE_CURVE ( 'NONE', #9423, #17658, #10804, .T. ) ;
#19172=LINE ( 'NONE', #5144, #4524 ) ;
#19189=EDGE_LOOP ( 'NONE', ( #2900, #8414, #15523, #20554 ) ) ;
#19212=DIRECTION ( 'NONE',  ( 0.000000000000000000, 1.000000000000000000, -2.999999999999999839E-15 ) ) ;
#19238=ORIENTED_EDGE ( 'NONE', *, *, #24901, .T. ) ;
#19268=ORIENTED_EDGE ( 'NONE', *, *, #21220, .F. ) ;
#19299=LINE ( 'NONE', #5270, #6655 ) ;
#19312=ADVANCED_FACE ( 'NONE', ( #17502 ), #9652, .F. ) ;
#19367=EDGE_LOOP ( 'NONE', ( #5180, #6917, #8336, #22682, #15583, #5970, #2711, #22435, #22577, #14291, #19268, #20806 ) ) ;
#19375=PRODUCT ( 'Staple Pusher', 'Staple Pusher', '', ( #7764 ) ) ;
#19394=ADVANCED_FACE ( 'NONE', ( #2141 ), #2397, .F. ) ;
#19398=ORIENTED_EDGE ( 'NONE', *, *, #15153, .T. ) ;
#19427=DIRECTION ( 'NONE',  ( 0.000000000000000000, -1.000000000000000000, 2.999999999999999839E-15 ) ) ;
#19517=ORIENTED_EDGE ( 'NONE', *, *, #6928, .T. ) ;
#19589=CARTESIAN_POINT ( 'NONE',  ( 42.81606138205700063, 16.19123852234699967, 69.30501292736995822 ) ) ;
#19644=EDGE_CURVE ( 'NONE', #467, #4421, #13468, .T. ) ;
#19648=VECTOR ( 'NONE', #9814, 1000.000000000000000 ) ;
#19678=VERTEX_POINT ( 'NONE', #21079 ) ;
#19686=VECTOR ( 'NONE', #17210, 1000.000000000000000 ) ;
#19687=ORIENTED_EDGE ( 'NONE', *, *, #22004, .T. ) ;
#19741=ORIENTED_EDGE ( 'NONE', *, *, #2404, .T. ) ;
#19761=CARTESIAN_POINT ( 'NONE',  ( 35.81606138205700063, 5.191238522346999673, 69.30501292736998664 ) ) ;
#19767=ORIENTED_EDGE ( 'NONE', *, *, #19104, .F. ) ;
#19772=ORIENTED_EDGE ( 'NONE', *, *, #20895, .T. ) ;
#19828=VECTOR ( 'NONE', #17128, 1000.000000000000000 ) ;
#19870=VECTOR ( 'NONE', #16769, 1000.000000000000000 ) ;
#19878=CARTESIAN_POINT ( 'NONE',  ( 40.81606138205700063, 5.191238522346999673, 69.30501292736998664 ) ) ;
#19885=CARTESIAN_POINT ( 'NONE',  ( 32.81606138205700773, 2.191238522347000117, 69.30501292737000085 ) ) ;
#19906=FACE_OUTER_BOUND ( 'NONE', #6115, .T. ) ;
#19925=CYLINDRICAL_SURFACE ( 'NONE', #10573, 0.5000000000000004441 ) ;
#19958=EDGE_CURVE ( 'NONE', #19015, #1986, #22076, .T. ) ;
#19995=CARTESIAN_POINT ( 'NONE',  ( 38.31606138205700063, 12.69123852234700678, 71.30501292736997243 ) ) ;
#20021=DIRECTION ( 'NONE',  ( 0.000000000000000000, 1.000000000000000000, -2.999999999999999839E-15 ) ) ;
#20038=LINE ( 'NONE', #16416, #13278 ) ;
#20078=CARTESIAN_POINT ( 'NONE',  ( 40.31606138205700063, 8.691238522346997897, 68.80501292736998664 ) ) ;
#20081=EDGE_CURVE ( 'NONE', #7071, #10377, #8943, .T. ) ;
#20083=DIRECTION ( 'NONE',  ( 0.000000000000000000, 1.000000000000000000, -2.999999999999999839E-15 ) ) ;
#20108=CARTESIAN_POINT ( 'NONE',  ( 35.81606138205700063, 5.691238522347000561, 69.30501292736998664 ) ) ;
#20134=CARTESIAN_POINT ( 'NONE',  ( 42.68042513965293949, 15.19123852234700323, 70.30501292736995822 ) ) ;
#20189=DIRECTION ( 'NONE',  ( 1.000000000000000000, 0.000000000000000000, -0.000000000000000000 ) ) ;
#20244=ORIENTED_EDGE ( 'NONE', *, *, #17518, .F. ) ;
#20260=LINE ( 'NONE', #19885, #17005 ) ;
#20283=EDGE_CURVE ( 'NONE', #6369, #3058, #7391, .T. ) ;
#20292=CARTESIAN_POINT ( 'NONE',  ( 36.52316816324354676, 8.484131741160446438, 65.30501292736998664 ) ) ;
#20294=CARTESIAN_POINT ( 'NONE',  ( 40.81606138205700063, 5.191238522346999673, 69.30501292736998664 ) ) ;
#20331=CARTESIAN_POINT ( 'NONE',  ( 33.81606138205700063, 16.19123852234699967, 69.30501292736995822 ) ) ;
#20363=CARTESIAN_POINT ( 'NONE',  ( 38.31606138205700063, 12.69123852234700678, 71.30501292736997243 ) ) ;
#20385=DIRECTION ( 'NONE',  ( 0.000000000000000000, -1.000000000000000000, 0.000000000000000000 ) ) ;
#20443=DIRECTION ( 'NONE',  ( 0.000000000000000000, -1.000000000000000000, 2.999999999999999839E-15 ) ) ;
#20454=CARTESIAN_POINT ( 'NONE',  ( 33.81606138205700063, 2.191238522347013440, 73.80501292737000085 ) ) ;
#20474=CARTESIAN_POINT ( 'NONE',  ( 42.81606138205700063, 22.19123852234699967, 69.30501292736994401 ) ) ;
#20554=ORIENTED_EDGE ( 'NONE', *, *, #1906, .F. ) ;
#20572=CARTESIAN_POINT ( 'NONE',  ( 38.31606138205700063, 15.19123852234700500, 71.30501292736995822 ) ) ;
#20638=DIRECTION ( 'NONE',  ( 0.000000000000000000, -1.000000000000000000, 2.999999999999999839E-15 ) ) ;
#20667=EDGE_LOOP ( 'NONE', ( #19767, #1829, #12032, #4683 ) ) ;
#20673=ORIENTED_EDGE ( 'NONE', *, *, #12439, .T. ) ;
#20683=ORIENTED_EDGE ( 'NONE', *, *, #25045, .F. ) ;
#20689=AXIS2_PLACEMENT_3D ( 'NONE', #18032, #16080, #23929 ) ;
#20772=VECTOR ( 'NONE', #19212, 1000.000000000000000 ) ;
#20806=ORIENTED_EDGE ( 'NONE', *, *, #6576, .F. ) ;
#20814=ORIENTED_EDGE ( 'NONE', *, *, #23554, .F. ) ;
#20821=ORIENTED_EDGE ( 'NONE', *, *, #7774, .T. ) ;
#20823=DIRECTION ( 'NONE',  ( -1.000000000000000000, 0.000000000000000000, 0.000000000000000000 ) ) ;
#20831=CARTESIAN_POINT ( 'NONE',  ( 32.81606138205700773, 22.19123852234699967, 69.30501292736994401 ) ) ;
#20865=AXIS2_PLACEMENT_3D ( 'NONE', #23119, #3425, #1981 ) ;
#20879=ORIENTED_EDGE ( 'NONE', *, *, #650, .T. ) ;
#20891=VERTEX_POINT ( 'NONE', #22928 ) ;
#20895=EDGE_CURVE ( 'NONE', #9681, #22879, #732, .T. ) ;
#20896=CARTESIAN_POINT ( 'NONE',  ( 40.31606138205700063, 5.191238522346998785, 68.80501292736998664 ) ) ;
#20904=CARTESIAN_POINT ( 'NONE',  ( 32.81606138205700773, 2.191238522347000117, 69.30501292737000085 ) ) ;
#20906=PLANE ( 'NONE',  #17624 ) ;
#20936=EDGE_CURVE ( 'NONE', #17636, #22981, #11998, .T. ) ;
#20946=( BOUNDED_CURVE ( )  B_SPLINE_CURVE ( 3, ( #1911, #7864, #25349, #5661 ),
 .UNSPECIFIED., .F., .T. ) 
 B_SPLINE_CURVE_WITH_KNOTS ( ( 4, 4 ),
 ( 3.141592653589795336, 4.712388980384689674 ),
 .UNSPECIFIED. ) 
 CURVE ( )  GEOMETRIC_REPRESENTATION_ITEM ( )  RATIONAL_B_SPLINE_CURVE ( ( 1.000000000000000000, 0.8047378541243649375, 0.8047378541243649375, 1.000000000000000000 ) ) 
 REPRESENTATION_ITEM ( '' )  );
#20953=FILL_AREA_STYLE ('',( #15694 ) ) ;
#20960=CIRCLE ( 'NONE', #25026, 1.000000000000000888 ) ;
#20964=ORIENTED_EDGE ( 'NONE', *, *, #23554, .T. ) ;
#20986=EDGE_LOOP ( 'NONE', ( #21855, #18643, #1313, #13206 ) ) ;
#20995=ORIENTED_EDGE ( 'NONE', *, *, #16508, .T. ) ;
#21079=CARTESIAN_POINT ( 'NONE',  ( 36.31606138205700063, 5.691238522346998785, 68.80501292736998664 ) ) ;
#21093=FACE_BOUND ( 'NONE', #6924, .T. ) ;
#21101=CARTESIAN_POINT ( 'NONE',  ( 40.31606138205700063, 5.691238522346989903, 65.80501292736998664 ) ) ;
#21117=AXIS2_PLACEMENT_3D ( 'NONE', #18204, #8541, #16127 ) ;
#21140=ORIENTED_EDGE ( 'NONE', *, *, #593, .F. ) ;
#21143=( BOUNDED_CURVE ( )  B_SPLINE_CURVE ( 3, ( #22214, #20292, #2627, #2742 ),
 .UNSPECIFIED., .F., .T. ) 
 B_SPLINE_CURVE_WITH_KNOTS ( ( 4, 4 ),
 ( 1.570796326794895004, 3.141592653589795336 ),
 .UNSPECIFIED. ) 
 CURVE ( )  GEOMETRIC_REPRESENTATION_ITEM ( )  RATIONAL_B_SPLINE_CURVE ( ( 1.000000000000000000, 0.8047378541243649375, 0.8047378541243649375, 1.000000000000000000 ) ) 
 REPRESENTATION_ITEM ( '' )  );
#21168=FACE_OUTER_BOUND ( 'NONE', #6416, .T. ) ;
#21207=VECTOR ( 'NONE', #14670, 1000.000000000000000 ) ;
#21220=EDGE_CURVE ( 'NONE', #10160, #2724, #19172, .T. ) ;
#21224=CARTESIAN_POINT ( 'NONE',  ( 32.81606138205700773, 2.191238522347000117, 69.30501292737000085 ) ) ;
#21228=DIRECTION ( 'NONE',  ( 0.000000000000000000, -1.000000000000000000, 2.999999999999999839E-15 ) ) ;
#21236=ORIENTED_EDGE ( 'NONE', *, *, #6319, .T. ) ;
#21257=ADVANCED_FACE ( 'NONE', ( #19906 ), #18109, .F. ) ;
#21270=LINE ( 'NONE', #1930, #19648 ) ;
#21375=SHAPE_REPRESENTATION_RELATIONSHIP ( 'NONE' , 'NONE' ,  #15514, #6771 ) ;
#21455=ORIENTED_EDGE ( 'NONE', *, *, #13023, .F. ) ;
#21481=DIRECTION ( 'NONE',  ( 1.000000000000000000, 0.000000000000000000, -0.000000000000000000 ) ) ;
#21557=ORIENTED_EDGE ( 'NONE', *, *, #22175, .F. ) ;
#21649=DIRECTION ( 'NONE',  ( 0.000000000000000000, 1.000000000000000000, -2.999999999999999839E-15 ) ) ;
#21660=DIRECTION ( 'NONE',  ( 0.000000000000000000, 1.000000000000000000, -2.999999999999999839E-15 ) ) ;
#21742=CARTESIAN_POINT ( 'NONE',  ( 40.31606138205700063, 5.691238522346988127, 65.30501292736998664 ) ) ;
#21757=ADVANCED_FACE ( 'NONE', ( #17688 ), #12159, .F. ) ;
#21763=CARTESIAN_POINT ( 'NONE',  ( 32.81606138205700773, 2.191238522347000117, 69.30501292737000085 ) ) ;
#21769=CARTESIAN_POINT ( 'NONE',  ( 40.52316816324353965, 8.898345303533549355, 69.30501292736998664 ) ) ;
#21826=VERTEX_POINT ( 'NONE', #8533 ) ;
#21855=ORIENTED_EDGE ( 'NONE', *, *, #14600, .F. ) ;
#21879=STYLED_ITEM ( 'NONE', ( #1936 ), #17330 ) ;
#21892=FACE_OUTER_BOUND ( 'NONE', #1216, .T. ) ;
#21905=ORIENTED_EDGE ( 'NONE', *, *, #15631, .F. ) ;
#22002=FACE_OUTER_BOUND ( 'NONE', #23628, .T. ) ;
#22004=EDGE_CURVE ( 'NONE', #13614, #22981, #20960, .T. ) ;
#22019=ORIENTED_EDGE ( 'NONE', *, *, #23492, .F. ) ;
#22076=LINE ( 'NONE', #17851, #3237 ) ;
#22098=AXIS2_PLACEMENT_3D ( 'NONE', #16549, #3279, #6894 ) ;
#22114=DIRECTION ( 'NONE',  ( 0.000000000000000000, -1.000000000000000000, 2.999999999999999839E-15 ) ) ;
#22175=EDGE_CURVE ( 'NONE', #16802, #6235, #4500, .T. ) ;
#22214=CARTESIAN_POINT ( 'NONE',  ( 36.81606138205700063, 8.191238522346989015, 65.30501292736998664 ) ) ;
#22231=VERTEX_POINT ( 'NONE', #1001 ) ;
#22298=VECTOR ( 'NONE', #858, 1000.000000000000000 ) ;
#22360=ORIENTED_EDGE ( 'NONE', *, *, #16508, .F. ) ;
#22417=CARTESIAN_POINT ( 'NONE',  ( 40.31606138205700063, 5.691238522346998785, 68.80501292736998664 ) ) ;
#22435=ORIENTED_EDGE ( 'NONE', *, *, #19644, .T. ) ;
#22440=EDGE_LOOP ( 'NONE', ( #17713, #20244, #14491, #1007 ) ) ;
#22448=CARTESIAN_POINT ( 'NONE',  ( 32.81606138205700773, 22.19123852234699967, 69.30501292736994401 ) ) ;
#22502=VECTOR ( 'NONE', #17715, 1000.000000000000000 ) ;
#22523=ORIENTED_EDGE ( 'NONE', *, *, #18787, .T. ) ;
#22537=DIRECTION ( 'NONE',  ( 1.000000000000000000, 0.000000000000000000, 0.000000000000000000 ) ) ;
#22538=EDGE_LOOP ( 'NONE', ( #12409, #20964, #11717, #12219 ) ) ;
#22564=CARTESIAN_POINT ( 'NONE',  ( 39.81606138205699352, 6.191238522346988127, 65.30501292736998664 ) ) ;
#22568=CARTESIAN_POINT ( 'NONE',  ( 33.81606138205700063, 2.191238522347003226, 70.30501292737000085 ) ) ;
#22575=FACE_OUTER_BOUND ( 'NONE', #8058, .T. ) ;
#22577=ORIENTED_EDGE ( 'NONE', *, *, #2184, .T. ) ;
#22625=ORIENTED_EDGE ( 'NONE', *, *, #250, .F. ) ;
#22682=ORIENTED_EDGE ( 'NONE', *, *, #900, .F. ) ;
#22694=LINE ( 'NONE', #7244, #19870 ) ;
#22757=VECTOR ( 'NONE', #13624, 1000.000000000000000 ) ;
#22779=EDGE_CURVE ( 'NONE', #22879, #22231, #24039, .T. ) ;
#22806=CARTESIAN_POINT ( 'NONE',  ( 33.81606138205700063, 15.19123852234700323, 70.30501292736995822 ) ) ;
#22858=EDGE_CURVE ( 'NONE', #14577, #4754, #8857, .T. ) ;
#22879=VERTEX_POINT ( 'NONE', #16434 ) ;
#22928=CARTESIAN_POINT ( 'NONE',  ( 35.81606138205700063, 5.191238522346999673, 69.30501292736998664 ) ) ;
#22942=LINE ( 'NONE', #19589, #18010 ) ;
#22964=CARTESIAN_POINT ( 'NONE',  ( 43.81606138205700063, 2.191238522347000117, 69.30501292737000085 ) ) ;
#22981=VERTEX_POINT ( 'NONE', #11679 ) ;
#23037=VECTOR ( 'NONE', #23183, 1000.000000000000000 ) ;
#23119=CARTESIAN_POINT ( 'NONE',  ( 43.81606138205700063, 2.191238522347003226, 70.30501292737000085 ) ) ;
#23121=( NAMED_UNIT ( * ) SI_UNIT ( $, .STERADIAN. ) SOLID_ANGLE_UNIT ( ) );
#23122=ORIENTED_EDGE ( 'NONE', *, *, #24052, .T. ) ;
#23141=LINE ( 'NONE', #21101, #22757 ) ;
#23162=LINE ( 'NONE', #3583, #2622 ) ;
#23183=DIRECTION ( 'NONE',  ( 1.445602896647339903E-16, -1.000000000000000000, 2.999999999999999839E-15 ) ) ;
#23192=CARTESIAN_POINT ( 'NONE',  ( 33.81606138205700063, 15.19123852234701388, 73.80501292736995822 ) ) ;
#23210=PRODUCT_DEFINITION_FORMATION_WITH_SPECIFIED_SOURCE ( 'ANY', '', #19375, .NOT_KNOWN. ) ;
#23212=EDGE_CURVE ( 'NONE', #4421, #16465, #10239, .T. ) ;
#23238=ORIENTED_EDGE ( 'NONE', *, *, #4139, .T. ) ;
#23294=( LENGTH_UNIT ( ) NAMED_UNIT ( * ) SI_UNIT ( .MILLI., .METRE. ) );
#23480=FACE_OUTER_BOUND ( 'NONE', #5623, .T. ) ;
#23492=EDGE_CURVE ( 'NONE', #17658, #19678, #15331, .T. ) ;
#23510=ORIENTED_EDGE ( 'NONE', *, *, #3205, .F. ) ;
#23512=LINE ( 'NONE', #9636, #904 ) ;
#23529=VECTOR ( 'NONE', #15539, 1000.000000000000000 ) ;
#23554=EDGE_CURVE ( 'NONE', #1986, #4892, #11485, .T. ) ;
#23567=CARTESIAN_POINT ( 'NONE',  ( 36.31606138205700063, 5.691238522346998785, 68.80501292736998664 ) ) ;
#23576=CARTESIAN_POINT ( 'NONE',  ( 38.31606138205700063, 16.19123852234700678, 71.30501292736995822 ) ) ;
#23585=( NAMED_UNIT ( * ) SI_UNIT ( $, .STERADIAN. ) SOLID_ANGLE_UNIT ( ) );
#23623=( BOUNDED_CURVE ( )  B_SPLINE_CURVE ( 3, ( #19878, #2217, #14330, #10097 ),
 .UNSPECIFIED., .F., .T. ) 
 B_SPLINE_CURVE_WITH_KNOTS ( ( 4, 4 ),
 ( 1.570796326794895004, 3.141592653589795336 ),
 .UNSPECIFIED. ) 
 CURVE ( )  GEOMETRIC_REPRESENTATION_ITEM ( )  RATIONAL_B_SPLINE_CURVE ( ( 1.000000000000000000, 0.8047378541243649375, 0.8047378541243649375, 1.000000000000000000 ) ) 
 REPRESENTATION_ITEM ( '' )  );
#23628=EDGE_LOOP ( 'NONE', ( #15139, #10368, #13390, #16815 ) ) ;
#23668=CARTESIAN_POINT ( 'NONE',  ( 32.81606138205700773, 2.191238522347000117, 69.30501292737000085 ) ) ;
#23690=ORIENTED_EDGE ( 'NONE', *, *, #18983, .F. ) ;
#23708=DIRECTION ( 'NONE',  ( 0.000000000000000000, -2.999999999999999839E-15, -1.000000000000000000 ) ) ;
#23775=DIRECTION ( 'NONE',  ( 0.000000000000000000, 1.000000000000000000, -2.999999999999999839E-15 ) ) ;
#23792=ORIENTED_EDGE ( 'NONE', *, *, #15572, .T. ) ;
#23809=DIRECTION ( 'NONE',  ( 0.000000000000000000, 1.000000000000000000, 0.000000000000000000 ) ) ;
#23829=CYLINDRICAL_SURFACE ( 'NONE', #15228, 0.5000000000000004441 ) ;
#23831=CYLINDRICAL_SURFACE ( 'NONE', #3347, 1.000000000000000888 ) ;
#23899=CARTESIAN_POINT ( 'NONE',  ( 43.81606138205700063, 6.191238522346989903, 65.80501292736998664 ) ) ;
#23910=DIRECTION ( 'NONE',  ( 1.000000000000000000, 0.000000000000000000, -0.000000000000000000 ) ) ;
#23929=DIRECTION ( 'NONE',  ( 1.000000000000000000, 0.000000000000000000, 0.000000000000000000 ) ) ;
#23933=DIRECTION ( 'NONE',  ( -1.000000000000000000, 0.000000000000000000, 0.000000000000000000 ) ) ;
#23959=CARTESIAN_POINT ( 'NONE',  ( 36.10895460087045450, 8.898345303533549355, 69.30501292736998664 ) ) ;
#23966=CARTESIAN_POINT ( 'NONE',  ( 36.31606138205700063, 8.691238522346997897, 68.80501292736998664 ) ) ;
#23990=EDGE_LOOP ( 'NONE', ( #14620, #20879, #14460, #19398 ) ) ;
#23998=( GEOMETRIC_REPRESENTATION_CONTEXT ( 3 ) GLOBAL_UNCERTAINTY_ASSIGNED_CONTEXT ( ( #19055 ) ) GLOBAL_UNIT_ASSIGNED_CONTEXT ( ( #13232, #3295, #23121 ) ) REPRESENTATION_CONTEXT ( 'NONE', 'WORKASPACE' ) );
#24019=CARTESIAN_POINT ( 'NONE',  ( 43.81606138205700063, 22.19123852234699967, 69.30501292736994401 ) ) ;
#24039=LINE ( 'NONE', #2652, #13562 ) ;
#24052=EDGE_CURVE ( 'NONE', #9423, #4892, #16489, .T. ) ;
#24082=FACE_OUTER_BOUND ( 'NONE', #1983, .T. ) ;
#24084=DIRECTION ( 'NONE',  ( -1.000000000000000000, 0.000000000000000000, 0.000000000000000000 ) ) ;
#24144=LINE ( 'NONE', #10519, #6465 ) ;
#24239=DIRECTION ( 'NONE',  ( 0.000000000000000000, 2.999999999999999839E-15, 1.000000000000000000 ) ) ;
#24270=ADVANCED_FACE ( 'NONE', ( #10536 ), #12218, .F. ) ;
#24293=VECTOR ( 'NONE', #15417, 1000.000000000000000 ) ;
#24364=CARTESIAN_POINT ( 'NONE',  ( 33.81606138205700063, 22.19123852234703520, 80.30501292736994401 ) ) ;
#24386=VECTOR ( 'NONE', #11382, 1000.000000000000000 ) ;
#24401=ORIENTED_EDGE ( 'NONE', *, *, #13023, .T. ) ;
#24419=DIRECTION ( 'NONE',  ( -1.000000000000000000, 0.000000000000000000, 0.000000000000000000 ) ) ;
#24484=DIRECTION ( 'NONE',  ( -1.000000000000000000, 0.000000000000000000, 0.000000000000000000 ) ) ;
#24499=ADVANCED_FACE ( 'NONE', ( #3035 ), #10912, .F. ) ;
#24518=CARTESIAN_POINT ( 'NONE',  ( 39.81606138205699352, 8.191238522346989015, 65.30501292736998664 ) ) ;
#24537=VECTOR ( 'NONE', #4798, 1000.000000000000000 ) ;
#24566=( BOUNDED_CURVE ( )  B_SPLINE_CURVE ( 3, ( #16107, #2317, #23959, #6455 ),
 .UNSPECIFIED., .F., .T. ) 
 B_SPLINE_CURVE_WITH_KNOTS ( ( 4, 4 ),
 ( 0.000000000000000000, 1.570796326794895004 ),
 .UNSPECIFIED. ) 
 CURVE ( )  GEOMETRIC_REPRESENTATION_ITEM ( )  RATIONAL_B_SPLINE_CURVE ( ( 1.000000000000000000, 0.8047378541243649375, 0.8047378541243649375, 1.000000000000000000 ) ) 
 REPRESENTATION_ITEM ( '' )  );
#24602=ORIENTED_EDGE ( 'NONE', *, *, #650, .F. ) ;
#24634=ORIENTED_EDGE ( 'NONE', *, *, #231, .T. ) ;
#24636=CARTESIAN_POINT ( 'NONE',  ( 43.81606138205700063, 2.191238522347013440, 73.80501292737000085 ) ) ;
#24675=ORIENTED_EDGE ( 'NONE', *, *, #12866, .T. ) ;
#24698=ORIENTED_EDGE ( 'NONE', *, *, #6928, .F. ) ;
#24716=VECTOR ( 'NONE', #1998, 1000.000000000000000 ) ;
#24721=ORIENTED_EDGE ( 'NONE', *, *, #20895, .F. ) ;
#24745=LINE ( 'NONE', #22448, #24537 ) ;
#24776=ORIENTED_EDGE ( 'NONE', *, *, #9264, .F. ) ;
#24861=ORIENTED_EDGE ( 'NONE', *, *, #22858, .F. ) ;
#24877=DIRECTION ( 'NONE',  ( -1.000000000000000000, 0.000000000000000000, 0.000000000000000000 ) ) ;
#24901=EDGE_CURVE ( 'NONE', #21826, #13614, #25051, .T. ) ;
#25026=AXIS2_PLACEMENT_3D ( 'NONE', #14958, #7233, #19085 ) ;
#25032=VECTOR ( 'NONE', #553, 1000.000000000000000 ) ;
#25045=EDGE_CURVE ( 'NONE', #3314, #4334, #6137, .T. ) ;
#25051=LINE ( 'NONE', #7820, #5398 ) ;
#25055=CIRCLE ( 'NONE', #383, 1.000000000000000888 ) ;
#25070=VERTEX_POINT ( 'NONE', #12329 ) ;
#25082=ORIENTED_EDGE ( 'NONE', *, *, #18851, .T. ) ;
#25097=ORIENTED_EDGE ( 'NONE', *, *, #20936, .F. ) ;
#25104=FACE_OUTER_BOUND ( 'NONE', #22538, .T. ) ;
#25119=CARTESIAN_POINT ( 'NONE',  ( 39.81606138205699352, 8.191238522346989015, 65.30501292736998664 ) ) ;
#25232=DIRECTION ( 'NONE',  ( -1.000000000000000000, 0.000000000000000000, 0.000000000000000000 ) ) ;
#25249=( LENGTH_UNIT ( ) NAMED_UNIT ( * ) SI_UNIT ( .MILLI., .METRE. ) );
#25326=CARTESIAN_POINT ( 'NONE',  ( 36.31606138205700063, 5.691238522346988127, 65.30501292736998664 ) ) ;
#25348=SURFACE_SIDE_STYLE ('',( #2293 ) ) ;
#25349=CARTESIAN_POINT ( 'NONE',  ( 36.52316816324354676, 5.898345303533535144, 65.30501292737000085 ) ) ;
#25354=ORIENTED_EDGE ( 'NONE', *, *, #15631, .T. ) ;
ENDSEC;
END-ISO-10303-21;
